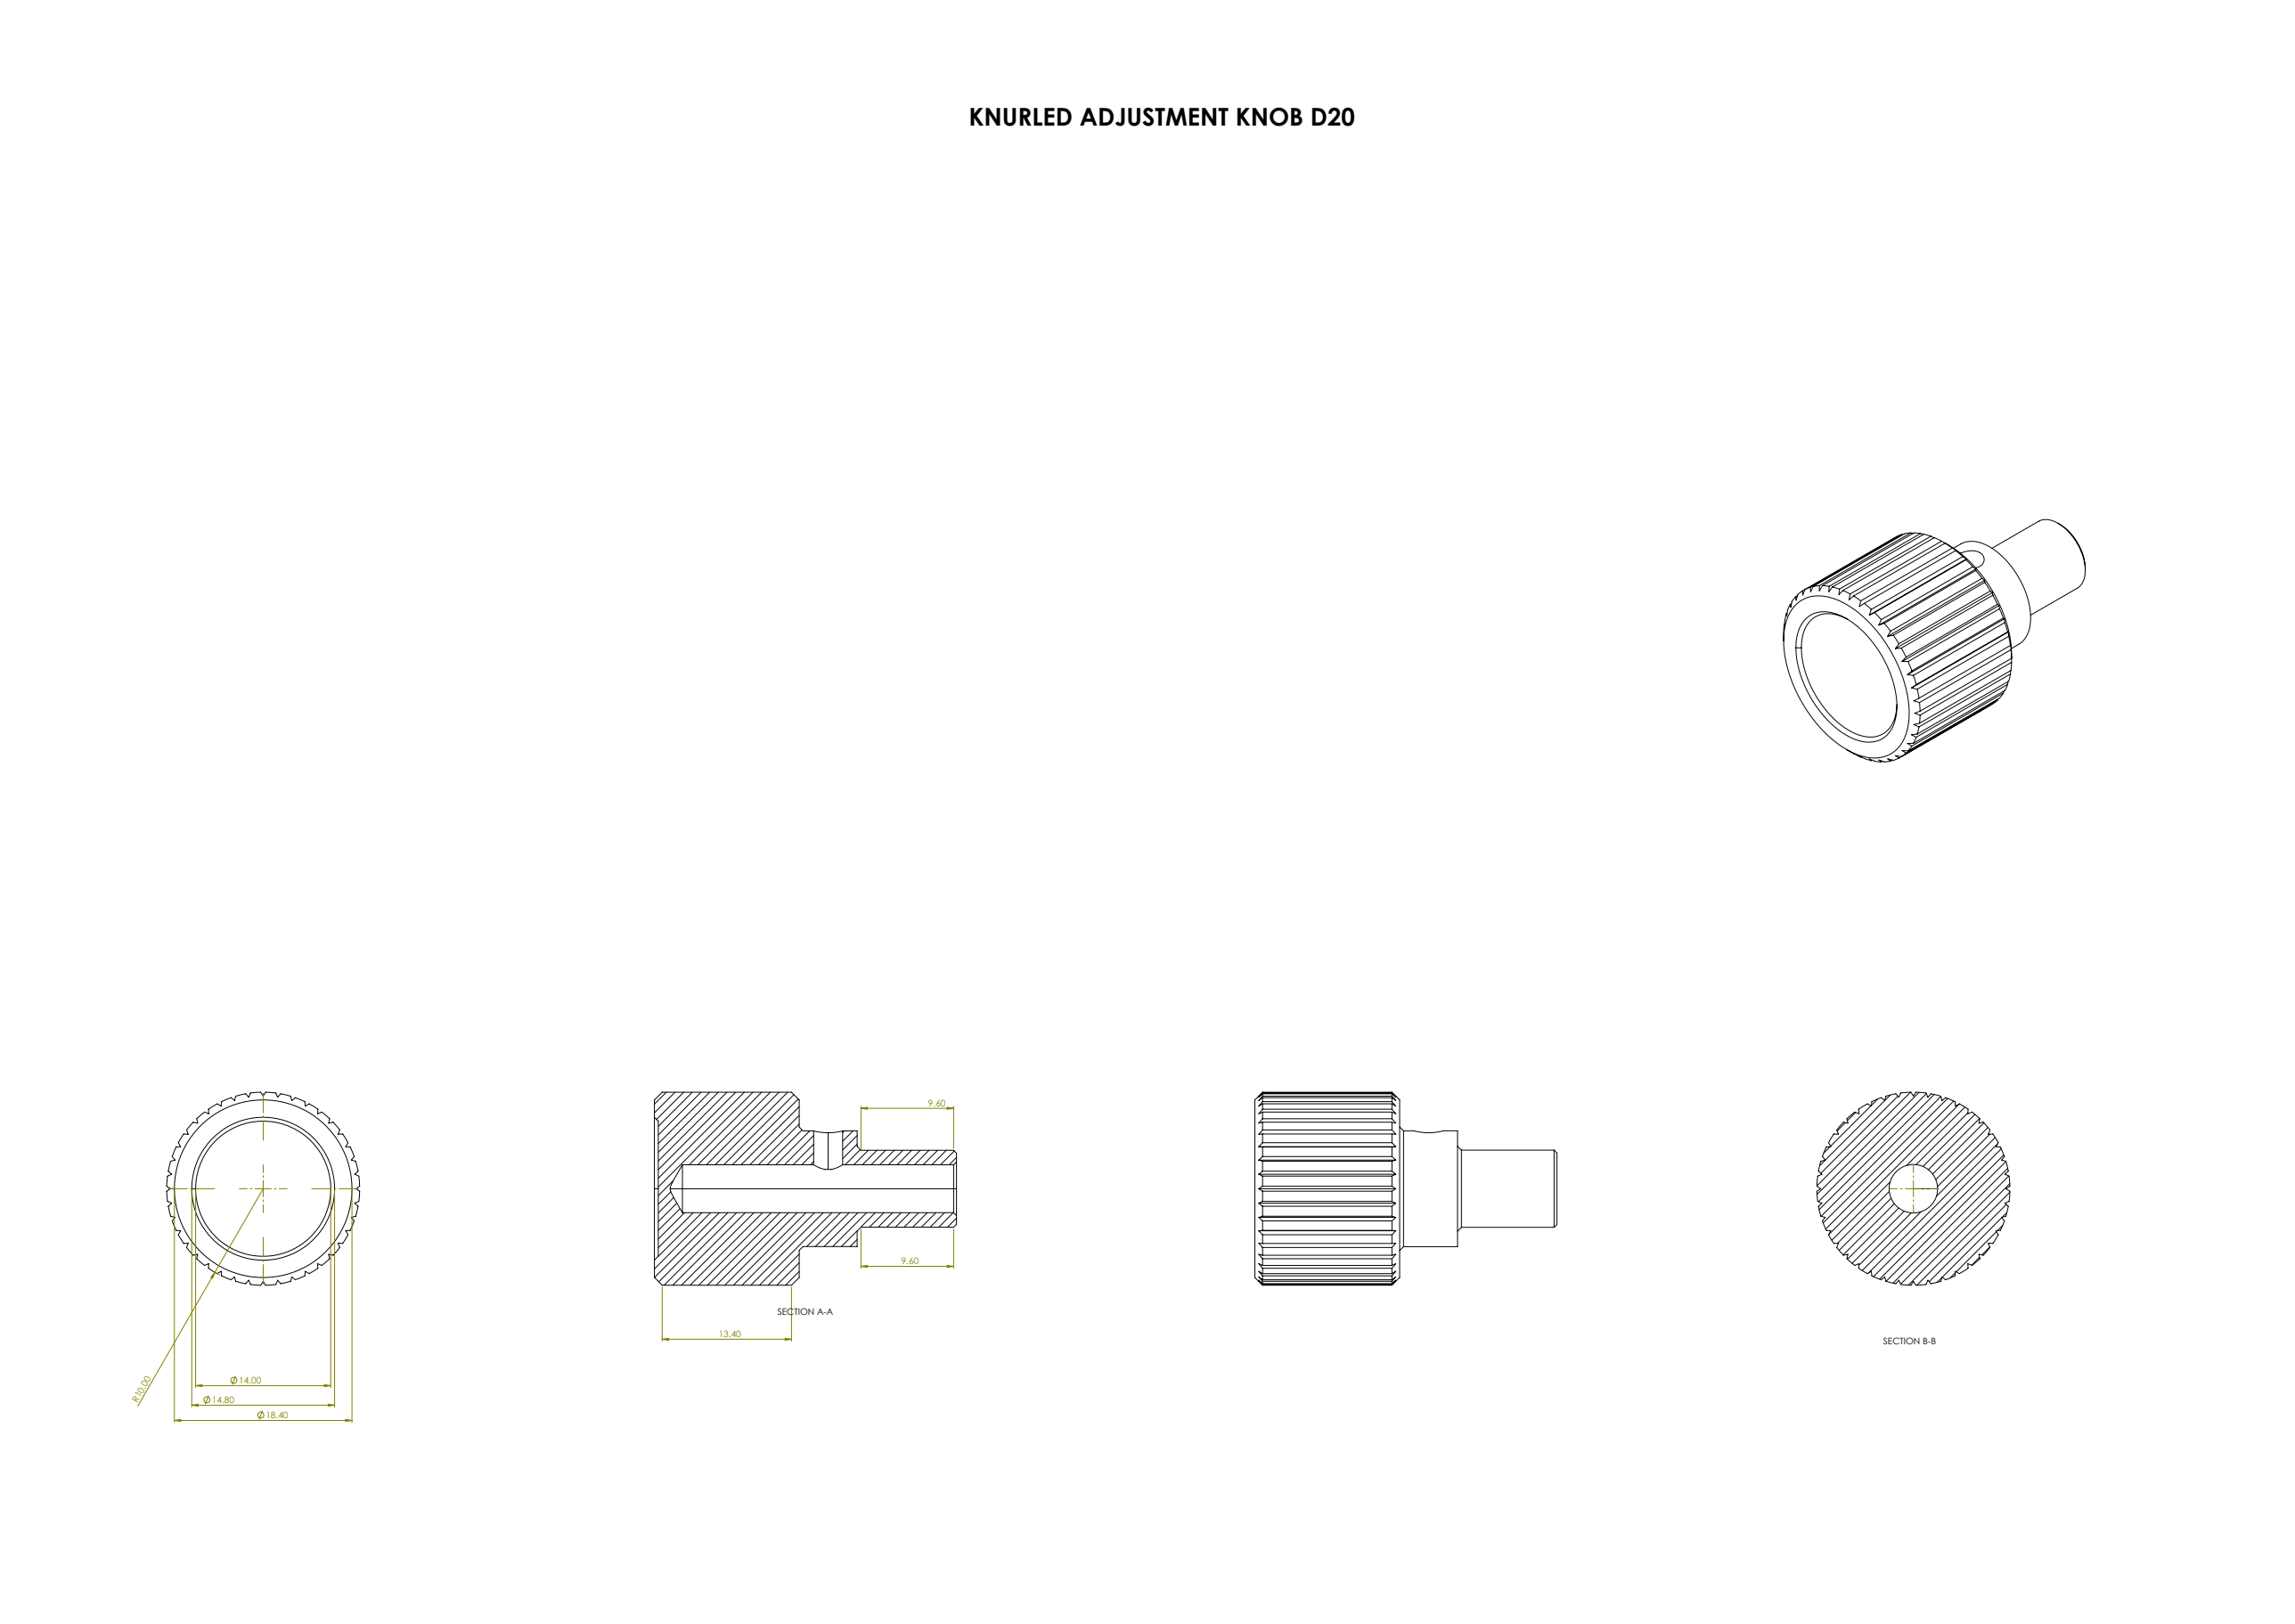
ISO-10303-21;
HEADER;
/* Generated by software containing ST-Developer
 * from STEP Tools, Inc. (www.steptools.com) 
 */

FILE_DESCRIPTION(
/* description */ (''),
/* implementation_level */ '2;1');

FILE_NAME(
/* name */ 'Knurled Adjustment Knob D20.step',
/* time_stamp */ '2026-10-05T09:57:53+05:00',
/* author */ (''),
/* organization */ (''),
/* preprocessor_version */ 'ST-DEVELOPER v20.2',
/* originating_system */ 'Autodesk Translation Framework v15.15.0.0',
/* authorisation */ '');

FILE_SCHEMA (('AUTOMOTIVE_DESIGN { 1 0 10303 214 3 1 1 }'));
ENDSEC;

DATA;
#10=MECHANICAL_DESIGN_GEOMETRIC_PRESENTATION_REPRESENTATION('',(#556),#113984);
#211=(
BOUNDED_CURVE()
B_SPLINE_CURVE(2,(#97814,#97815,#97816),.UNSPECIFIED.,.F.,.F.)
B_SPLINE_CURVE_WITH_KNOTS((3,3),(0.0639904841458714,0.1243156910283),
 .UNSPECIFIED.)
CURVE()
GEOMETRIC_REPRESENTATION_ITEM()
RATIONAL_B_SPLINE_CURVE((1.0006146198185,1.00059701757594,1.))
REPRESENTATION_ITEM('')
);
#212=(
BOUNDED_CURVE()
B_SPLINE_CURVE(2,(#97820,#97821,#97822),.UNSPECIFIED.,.F.,.F.)
B_SPLINE_CURVE_WITH_KNOTS((3,3),(0.,0.0603252068824429),.UNSPECIFIED.)
CURVE()
GEOMETRIC_REPRESENTATION_ITEM()
RATIONAL_B_SPLINE_CURVE((1.,1.00059701758504,1.00061461982786))
REPRESENTATION_ITEM('')
);
#213=(
BOUNDED_CURVE()
B_SPLINE_CURVE(2,(#97826,#97827,#97828),.UNSPECIFIED.,.F.,.F.)
B_SPLINE_CURVE_WITH_KNOTS((3,3),(0.,0.0603252068824511),.UNSPECIFIED.)
CURVE()
GEOMETRIC_REPRESENTATION_ITEM()
RATIONAL_B_SPLINE_CURVE((1.,1.00059701757207,1.00061461981452))
REPRESENTATION_ITEM('')
);
#214=(
BOUNDED_CURVE()
B_SPLINE_CURVE(2,(#97831,#97832,#97833),.UNSPECIFIED.,.F.,.F.)
B_SPLINE_CURVE_WITH_KNOTS((3,3),(0.0639904841458541,0.124315691028304),
 .UNSPECIFIED.)
CURVE()
GEOMETRIC_REPRESENTATION_ITEM()
RATIONAL_B_SPLINE_CURVE((1.00061461982307,1.00059701758038,1.))
REPRESENTATION_ITEM('')
);
#215=(
BOUNDED_CURVE()
B_SPLINE_CURVE(2,(#97838,#97839,#97840),.UNSPECIFIED.,.F.,.F.)
B_SPLINE_CURVE_WITH_KNOTS((3,3),(0.,0.0603252068825254),.UNSPECIFIED.)
CURVE()
GEOMETRIC_REPRESENTATION_ITEM()
RATIONAL_B_SPLINE_CURVE((1.,1.00059701756463,1.00061461980685))
REPRESENTATION_ITEM('')
);
#216=(
BOUNDED_CURVE()
B_SPLINE_CURVE(2,(#97842,#97843,#97844),.UNSPECIFIED.,.F.,.F.)
B_SPLINE_CURVE_WITH_KNOTS((3,3),(0.0639904841458276,0.124315691028306),
 .UNSPECIFIED.)
CURVE()
GEOMETRIC_REPRESENTATION_ITEM()
RATIONAL_B_SPLINE_CURVE((1.00061461981098,1.00059701756864,1.))
REPRESENTATION_ITEM('')
);
#217=(
BOUNDED_CURVE()
B_SPLINE_CURVE(2,(#97848,#97849,#97850),.UNSPECIFIED.,.F.,.F.)
B_SPLINE_CURVE_WITH_KNOTS((3,3),(0.,0.0603252068824394),.UNSPECIFIED.)
CURVE()
GEOMETRIC_REPRESENTATION_ITEM()
RATIONAL_B_SPLINE_CURVE((1.,1.00059701757103,1.00061461981344))
REPRESENTATION_ITEM('')
);
#218=(
BOUNDED_CURVE()
B_SPLINE_CURVE(2,(#97852,#97853,#97854),.UNSPECIFIED.,.F.,.F.)
B_SPLINE_CURVE_WITH_KNOTS((3,3),(0.0639904841458415,0.124315691028305),
 .UNSPECIFIED.)
CURVE()
GEOMETRIC_REPRESENTATION_ITEM()
RATIONAL_B_SPLINE_CURVE((1.00061461981036,1.00059701756804,1.))
REPRESENTATION_ITEM('')
);
#219=(
BOUNDED_CURVE()
B_SPLINE_CURVE(2,(#97858,#97859,#97860),.UNSPECIFIED.,.F.,.F.)
B_SPLINE_CURVE_WITH_KNOTS((3,3),(0.,0.0603252068825714),.UNSPECIFIED.)
CURVE()
GEOMETRIC_REPRESENTATION_ITEM()
RATIONAL_B_SPLINE_CURVE((1.,1.00059701757132,1.00061461981374))
REPRESENTATION_ITEM('')
);
#220=(
BOUNDED_CURVE()
B_SPLINE_CURVE(2,(#97862,#97863,#97864),.UNSPECIFIED.,.F.,.F.)
B_SPLINE_CURVE_WITH_KNOTS((3,3),(0.0639904841458359,0.124315691028304),
 .UNSPECIFIED.)
CURVE()
GEOMETRIC_REPRESENTATION_ITEM()
RATIONAL_B_SPLINE_CURVE((1.00061461982205,1.00059701757939,1.))
REPRESENTATION_ITEM('')
);
#221=(
BOUNDED_CURVE()
B_SPLINE_CURVE(2,(#97868,#97869,#97870),.UNSPECIFIED.,.F.,.F.)
B_SPLINE_CURVE_WITH_KNOTS((3,3),(0.,0.0603252068824456),.UNSPECIFIED.)
CURVE()
GEOMETRIC_REPRESENTATION_ITEM()
RATIONAL_B_SPLINE_CURVE((1.,1.00059701756571,1.00061461980796))
REPRESENTATION_ITEM('')
);
#222=(
BOUNDED_CURVE()
B_SPLINE_CURVE(2,(#97872,#97873,#97874),.UNSPECIFIED.,.F.,.F.)
B_SPLINE_CURVE_WITH_KNOTS((3,3),(0.0639904841458113,0.124315691028305),
 .UNSPECIFIED.)
CURVE()
GEOMETRIC_REPRESENTATION_ITEM()
RATIONAL_B_SPLINE_CURVE((1.00061461980765,1.00059701756541,1.))
REPRESENTATION_ITEM('')
);
#223=(
BOUNDED_CURVE()
B_SPLINE_CURVE(2,(#97878,#97879,#97880),.UNSPECIFIED.,.F.,.F.)
B_SPLINE_CURVE_WITH_KNOTS((3,3),(0.,0.0603252068824822),.UNSPECIFIED.)
CURVE()
GEOMETRIC_REPRESENTATION_ITEM()
RATIONAL_B_SPLINE_CURVE((1.,1.00059701756982,1.0006146198122))
REPRESENTATION_ITEM('')
);
#224=(
BOUNDED_CURVE()
B_SPLINE_CURVE(2,(#97882,#97883,#97884),.UNSPECIFIED.,.F.,.F.)
B_SPLINE_CURVE_WITH_KNOTS((3,3),(0.0639904841458351,0.124315691028304),
 .UNSPECIFIED.)
CURVE()
GEOMETRIC_REPRESENTATION_ITEM()
RATIONAL_B_SPLINE_CURVE((1.0006146198107,1.00059701756837,1.))
REPRESENTATION_ITEM('')
);
#225=(
BOUNDED_CURVE()
B_SPLINE_CURVE(2,(#97888,#97889,#97890),.UNSPECIFIED.,.F.,.F.)
B_SPLINE_CURVE_WITH_KNOTS((3,3),(0.,0.0603252068824583),.UNSPECIFIED.)
CURVE()
GEOMETRIC_REPRESENTATION_ITEM()
RATIONAL_B_SPLINE_CURVE((1.,1.00059701757041,1.0006146198128))
REPRESENTATION_ITEM('')
);
#226=(
BOUNDED_CURVE()
B_SPLINE_CURVE(2,(#97892,#97893,#97894),.UNSPECIFIED.,.F.,.F.)
B_SPLINE_CURVE_WITH_KNOTS((3,3),(0.0639904841458709,0.124315691028304),
 .UNSPECIFIED.)
CURVE()
GEOMETRIC_REPRESENTATION_ITEM()
RATIONAL_B_SPLINE_CURVE((1.00061461981124,1.00059701756889,1.))
REPRESENTATION_ITEM('')
);
#227=(
BOUNDED_CURVE()
B_SPLINE_CURVE(2,(#97898,#97899,#97900),.UNSPECIFIED.,.F.,.F.)
B_SPLINE_CURVE_WITH_KNOTS((3,3),(0.,0.0603252068824821),.UNSPECIFIED.)
CURVE()
GEOMETRIC_REPRESENTATION_ITEM()
RATIONAL_B_SPLINE_CURVE((1.,1.0005970175711,1.00061461981351))
REPRESENTATION_ITEM('')
);
#228=(
BOUNDED_CURVE()
B_SPLINE_CURVE(2,(#97902,#97903,#97904),.UNSPECIFIED.,.F.,.F.)
B_SPLINE_CURVE_WITH_KNOTS((3,3),(0.0639904841458647,0.124315691028304),
 .UNSPECIFIED.)
CURVE()
GEOMETRIC_REPRESENTATION_ITEM()
RATIONAL_B_SPLINE_CURVE((1.00061461981158,1.00059701756922,1.))
REPRESENTATION_ITEM('')
);
#229=(
BOUNDED_CURVE()
B_SPLINE_CURVE(2,(#97908,#97909,#97910),.UNSPECIFIED.,.F.,.F.)
B_SPLINE_CURVE_WITH_KNOTS((3,3),(0.,0.0603252068825191),.UNSPECIFIED.)
CURVE()
GEOMETRIC_REPRESENTATION_ITEM()
RATIONAL_B_SPLINE_CURVE((1.,1.00059701757121,1.00061461981363))
REPRESENTATION_ITEM('')
);
#230=(
BOUNDED_CURVE()
B_SPLINE_CURVE(2,(#97912,#97913,#97914),.UNSPECIFIED.,.F.,.F.)
B_SPLINE_CURVE_WITH_KNOTS((3,3),(0.063990484145815,0.124315691028306),
 .UNSPECIFIED.)
CURVE()
GEOMETRIC_REPRESENTATION_ITEM()
RATIONAL_B_SPLINE_CURVE((1.00061461981174,1.00059701756938,1.))
REPRESENTATION_ITEM('')
);
#231=(
BOUNDED_CURVE()
B_SPLINE_CURVE(2,(#97918,#97919,#97920),.UNSPECIFIED.,.F.,.F.)
B_SPLINE_CURVE_WITH_KNOTS((3,3),(0.,0.0603252068824783),.UNSPECIFIED.)
CURVE()
GEOMETRIC_REPRESENTATION_ITEM()
RATIONAL_B_SPLINE_CURVE((1.,1.00059701757256,1.00061461981502))
REPRESENTATION_ITEM('')
);
#232=(
BOUNDED_CURVE()
B_SPLINE_CURVE(2,(#97922,#97923,#97924),.UNSPECIFIED.,.F.,.F.)
B_SPLINE_CURVE_WITH_KNOTS((3,3),(0.0639904841458416,0.124315691028306),
 .UNSPECIFIED.)
CURVE()
GEOMETRIC_REPRESENTATION_ITEM()
RATIONAL_B_SPLINE_CURVE((1.00061461981231,1.00059701756993,1.))
REPRESENTATION_ITEM('')
);
#233=(
BOUNDED_CURVE()
B_SPLINE_CURVE(2,(#97928,#97929,#97930),.UNSPECIFIED.,.F.,.F.)
B_SPLINE_CURVE_WITH_KNOTS((3,3),(0.,0.0603252068824794),.UNSPECIFIED.)
CURVE()
GEOMETRIC_REPRESENTATION_ITEM()
RATIONAL_B_SPLINE_CURVE((1.,1.00059701756815,1.00061461981048))
REPRESENTATION_ITEM('')
);
#234=(
BOUNDED_CURVE()
B_SPLINE_CURVE(2,(#97932,#97933,#97934),.UNSPECIFIED.,.F.,.F.)
B_SPLINE_CURVE_WITH_KNOTS((3,3),(0.0639904841457963,0.124315691028306),
 .UNSPECIFIED.)
CURVE()
GEOMETRIC_REPRESENTATION_ITEM()
RATIONAL_B_SPLINE_CURVE((1.00061461981017,1.00059701756786,1.))
REPRESENTATION_ITEM('')
);
#235=(
BOUNDED_CURVE()
B_SPLINE_CURVE(2,(#97938,#97939,#97940),.UNSPECIFIED.,.F.,.F.)
B_SPLINE_CURVE_WITH_KNOTS((3,3),(0.,0.0603252068824883),.UNSPECIFIED.)
CURVE()
GEOMETRIC_REPRESENTATION_ITEM()
RATIONAL_B_SPLINE_CURVE((1.,1.00059701756951,1.00061461981188))
REPRESENTATION_ITEM('')
);
#236=(
BOUNDED_CURVE()
B_SPLINE_CURVE(2,(#97942,#97943,#97944),.UNSPECIFIED.,.F.,.F.)
B_SPLINE_CURVE_WITH_KNOTS((3,3),(0.0639904841458018,0.124315691028305),
 .UNSPECIFIED.)
CURVE()
GEOMETRIC_REPRESENTATION_ITEM()
RATIONAL_B_SPLINE_CURVE((1.00061461980912,1.00059701756684,1.))
REPRESENTATION_ITEM('')
);
#237=(
BOUNDED_CURVE()
B_SPLINE_CURVE(2,(#97948,#97949,#97950),.UNSPECIFIED.,.F.,.F.)
B_SPLINE_CURVE_WITH_KNOTS((3,3),(0.,0.0603252068824852),.UNSPECIFIED.)
CURVE()
GEOMETRIC_REPRESENTATION_ITEM()
RATIONAL_B_SPLINE_CURVE((1.,1.00059701756809,1.00061461981042))
REPRESENTATION_ITEM('')
);
#238=(
BOUNDED_CURVE()
B_SPLINE_CURVE(2,(#97952,#97953,#97954),.UNSPECIFIED.,.F.,.F.)
B_SPLINE_CURVE_WITH_KNOTS((3,3),(0.0639904841458453,0.124315691028304),
 .UNSPECIFIED.)
CURVE()
GEOMETRIC_REPRESENTATION_ITEM()
RATIONAL_B_SPLINE_CURVE((1.0006146198128,1.00059701757041,1.))
REPRESENTATION_ITEM('')
);
#239=(
BOUNDED_CURVE()
B_SPLINE_CURVE(2,(#97958,#97959,#97960),.UNSPECIFIED.,.F.,.F.)
B_SPLINE_CURVE_WITH_KNOTS((3,3),(0.,0.06032520688249),.UNSPECIFIED.)
CURVE()
GEOMETRIC_REPRESENTATION_ITEM()
RATIONAL_B_SPLINE_CURVE((1.,1.00059701756971,1.00061461981208))
REPRESENTATION_ITEM('')
);
#240=(
BOUNDED_CURVE()
B_SPLINE_CURVE(2,(#97962,#97963,#97964),.UNSPECIFIED.,.F.,.F.)
B_SPLINE_CURVE_WITH_KNOTS((3,3),(0.0639904841458239,0.124315691028304),
 .UNSPECIFIED.)
CURVE()
GEOMETRIC_REPRESENTATION_ITEM()
RATIONAL_B_SPLINE_CURVE((1.0006146198114,1.00059701756905,1.))
REPRESENTATION_ITEM('')
);
#241=(
BOUNDED_CURVE()
B_SPLINE_CURVE(2,(#97968,#97969,#97970),.UNSPECIFIED.,.F.,.F.)
B_SPLINE_CURVE_WITH_KNOTS((3,3),(0.,0.0603252068824721),.UNSPECIFIED.)
CURVE()
GEOMETRIC_REPRESENTATION_ITEM()
RATIONAL_B_SPLINE_CURVE((1.,1.0005970175654,1.00061461980764))
REPRESENTATION_ITEM('')
);
#242=(
BOUNDED_CURVE()
B_SPLINE_CURVE(2,(#97972,#97973,#97974),.UNSPECIFIED.,.F.,.F.)
B_SPLINE_CURVE_WITH_KNOTS((3,3),(0.0639904841458158,0.124315691028305),
 .UNSPECIFIED.)
CURVE()
GEOMETRIC_REPRESENTATION_ITEM()
RATIONAL_B_SPLINE_CURVE((1.00061461980759,1.00059701756535,1.))
REPRESENTATION_ITEM('')
);
#243=(
BOUNDED_CURVE()
B_SPLINE_CURVE(2,(#97978,#97979,#97980),.UNSPECIFIED.,.F.,.F.)
B_SPLINE_CURVE_WITH_KNOTS((3,3),(0.,0.0603252068824717),.UNSPECIFIED.)
CURVE()
GEOMETRIC_REPRESENTATION_ITEM()
RATIONAL_B_SPLINE_CURVE((1.,1.00059701757901,1.00061461982166))
REPRESENTATION_ITEM('')
);
#244=(
BOUNDED_CURVE()
B_SPLINE_CURVE(2,(#97982,#97983,#97984),.UNSPECIFIED.,.F.,.F.)
B_SPLINE_CURVE_WITH_KNOTS((3,3),(0.063990484145796,0.124315691028302),
 .UNSPECIFIED.)
CURVE()
GEOMETRIC_REPRESENTATION_ITEM()
RATIONAL_B_SPLINE_CURVE((1.0006146198112,1.00059701756885,1.))
REPRESENTATION_ITEM('')
);
#245=(
BOUNDED_CURVE()
B_SPLINE_CURVE(2,(#97988,#97989,#97990),.UNSPECIFIED.,.F.,.F.)
B_SPLINE_CURVE_WITH_KNOTS((3,3),(0.,0.0603252068824572),.UNSPECIFIED.)
CURVE()
GEOMETRIC_REPRESENTATION_ITEM()
RATIONAL_B_SPLINE_CURVE((1.,1.00059701757014,1.00061461981252))
REPRESENTATION_ITEM('')
);
#246=(
BOUNDED_CURVE()
B_SPLINE_CURVE(2,(#97992,#97993,#97994),.UNSPECIFIED.,.F.,.F.)
B_SPLINE_CURVE_WITH_KNOTS((3,3),(0.0639904841458277,0.124315691028304),
 .UNSPECIFIED.)
CURVE()
GEOMETRIC_REPRESENTATION_ITEM()
RATIONAL_B_SPLINE_CURVE((1.00061461981263,1.00059701757024,1.))
REPRESENTATION_ITEM('')
);
#247=(
BOUNDED_CURVE()
B_SPLINE_CURVE(2,(#97998,#97999,#98000),.UNSPECIFIED.,.F.,.F.)
B_SPLINE_CURVE_WITH_KNOTS((3,3),(0.,0.0603252068824675),.UNSPECIFIED.)
CURVE()
GEOMETRIC_REPRESENTATION_ITEM()
RATIONAL_B_SPLINE_CURVE((1.,1.00059701756283,1.000614619805))
REPRESENTATION_ITEM('')
);
#248=(
BOUNDED_CURVE()
B_SPLINE_CURVE(2,(#98002,#98003,#98004),.UNSPECIFIED.,.F.,.F.)
B_SPLINE_CURVE_WITH_KNOTS((3,3),(0.0639904841458849,0.124315691028304),
 .UNSPECIFIED.)
CURVE()
GEOMETRIC_REPRESENTATION_ITEM()
RATIONAL_B_SPLINE_CURVE((1.00061461981573,1.00059701757326,1.))
REPRESENTATION_ITEM('')
);
#249=(
BOUNDED_CURVE()
B_SPLINE_CURVE(2,(#98008,#98009,#98010),.UNSPECIFIED.,.F.,.F.)
B_SPLINE_CURVE_WITH_KNOTS((3,3),(0.,0.0603252068824598),.UNSPECIFIED.)
CURVE()
GEOMETRIC_REPRESENTATION_ITEM()
RATIONAL_B_SPLINE_CURVE((1.,1.0005970175702,1.00061461981259))
REPRESENTATION_ITEM('')
);
#250=(
BOUNDED_CURVE()
B_SPLINE_CURVE(2,(#98012,#98013,#98014),.UNSPECIFIED.,.F.,.F.)
B_SPLINE_CURVE_WITH_KNOTS((3,3),(0.0639904841458239,0.124315691028304),
 .UNSPECIFIED.)
CURVE()
GEOMETRIC_REPRESENTATION_ITEM()
RATIONAL_B_SPLINE_CURVE((1.00061461981594,1.00059701757346,1.))
REPRESENTATION_ITEM('')
);
#251=(
BOUNDED_CURVE()
B_SPLINE_CURVE(2,(#98018,#98019,#98020),.UNSPECIFIED.,.F.,.F.)
B_SPLINE_CURVE_WITH_KNOTS((3,3),(0.,0.0603252068824849),.UNSPECIFIED.)
CURVE()
GEOMETRIC_REPRESENTATION_ITEM()
RATIONAL_B_SPLINE_CURVE((1.,1.00059701756587,1.00061461980812))
REPRESENTATION_ITEM('')
);
#252=(
BOUNDED_CURVE()
B_SPLINE_CURVE(2,(#98025,#98026,#98027),.UNSPECIFIED.,.F.,.F.)
B_SPLINE_CURVE_WITH_KNOTS((3,3),(0.0639904841458217,0.124315691028305),
 .UNSPECIFIED.)
CURVE()
GEOMETRIC_REPRESENTATION_ITEM()
RATIONAL_B_SPLINE_CURVE((1.00061461980612,1.00059701756392,1.))
REPRESENTATION_ITEM('')
);
#253=(
BOUNDED_CURVE()
B_SPLINE_CURVE(2,(#98031,#98032,#98033),.UNSPECIFIED.,.F.,.F.)
B_SPLINE_CURVE_WITH_KNOTS((3,3),(0.,0.060325206882456),.UNSPECIFIED.)
CURVE()
GEOMETRIC_REPRESENTATION_ITEM()
RATIONAL_B_SPLINE_CURVE((1.,1.00059701757113,1.00061461981354))
REPRESENTATION_ITEM('')
);
#254=(
BOUNDED_CURVE()
B_SPLINE_CURVE(2,(#98035,#98036,#98037),.UNSPECIFIED.,.F.,.F.)
B_SPLINE_CURVE_WITH_KNOTS((3,3),(0.0639904841458245,0.124315691028306),
 .UNSPECIFIED.)
CURVE()
GEOMETRIC_REPRESENTATION_ITEM()
RATIONAL_B_SPLINE_CURVE((1.00061461981538,1.00059701757292,1.))
REPRESENTATION_ITEM('')
);
#255=(
BOUNDED_CURVE()
B_SPLINE_CURVE(2,(#98041,#98042,#98043),.UNSPECIFIED.,.F.,.F.)
B_SPLINE_CURVE_WITH_KNOTS((3,3),(0.,0.0603252068824492),.UNSPECIFIED.)
CURVE()
GEOMETRIC_REPRESENTATION_ITEM()
RATIONAL_B_SPLINE_CURVE((1.,1.0005970175686,1.00061461981094))
REPRESENTATION_ITEM('')
);
#256=(
BOUNDED_CURVE()
B_SPLINE_CURVE(2,(#98045,#98046,#98047),.UNSPECIFIED.,.F.,.F.)
B_SPLINE_CURVE_WITH_KNOTS((3,3),(0.0639904841457976,0.124315691028306),
 .UNSPECIFIED.)
CURVE()
GEOMETRIC_REPRESENTATION_ITEM()
RATIONAL_B_SPLINE_CURVE((1.00061461981101,1.00059701756867,1.))
REPRESENTATION_ITEM('')
);
#257=(
BOUNDED_CURVE()
B_SPLINE_CURVE(2,(#98051,#98052,#98053),.UNSPECIFIED.,.F.,.F.)
B_SPLINE_CURVE_WITH_KNOTS((3,3),(0.,0.0603252068824974),.UNSPECIFIED.)
CURVE()
GEOMETRIC_REPRESENTATION_ITEM()
RATIONAL_B_SPLINE_CURVE((1.,1.00059701757075,1.00061461981315))
REPRESENTATION_ITEM('')
);
#258=(
BOUNDED_CURVE()
B_SPLINE_CURVE(2,(#98055,#98056,#98057),.UNSPECIFIED.,.F.,.F.)
B_SPLINE_CURVE_WITH_KNOTS((3,3),(0.0639904841458211,0.124315691028304),
 .UNSPECIFIED.)
CURVE()
GEOMETRIC_REPRESENTATION_ITEM()
RATIONAL_B_SPLINE_CURVE((1.00061461981339,1.00059701757099,1.))
REPRESENTATION_ITEM('')
);
#259=(
BOUNDED_CURVE()
B_SPLINE_CURVE(2,(#98061,#98062,#98063),.UNSPECIFIED.,.F.,.F.)
B_SPLINE_CURVE_WITH_KNOTS((3,3),(0.,0.0603252068824656),.UNSPECIFIED.)
CURVE()
GEOMETRIC_REPRESENTATION_ITEM()
RATIONAL_B_SPLINE_CURVE((1.,1.00059701757014,1.00061461981252))
REPRESENTATION_ITEM('')
);
#260=(
BOUNDED_CURVE()
B_SPLINE_CURVE(2,(#98065,#98066,#98067),.UNSPECIFIED.,.F.,.F.)
B_SPLINE_CURVE_WITH_KNOTS((3,3),(0.0639904841457857,0.124315691028306),
 .UNSPECIFIED.)
CURVE()
GEOMETRIC_REPRESENTATION_ITEM()
RATIONAL_B_SPLINE_CURVE((1.00061461980911,1.00059701756683,1.))
REPRESENTATION_ITEM('')
);
#261=(
BOUNDED_CURVE()
B_SPLINE_CURVE(2,(#98071,#98072,#98073),.UNSPECIFIED.,.F.,.F.)
B_SPLINE_CURVE_WITH_KNOTS((3,3),(0.,0.0603252068825302),.UNSPECIFIED.)
CURVE()
GEOMETRIC_REPRESENTATION_ITEM()
RATIONAL_B_SPLINE_CURVE((1.,1.00059701756736,1.00061461980966))
REPRESENTATION_ITEM('')
);
#262=(
BOUNDED_CURVE()
B_SPLINE_CURVE(2,(#98075,#98076,#98077),.UNSPECIFIED.,.F.,.F.)
B_SPLINE_CURVE_WITH_KNOTS((3,3),(0.0639904841458149,0.124315691028305),
 .UNSPECIFIED.)
CURVE()
GEOMETRIC_REPRESENTATION_ITEM()
RATIONAL_B_SPLINE_CURVE((1.00061461980823,1.00059701756597,1.))
REPRESENTATION_ITEM('')
);
#263=(
BOUNDED_CURVE()
B_SPLINE_CURVE(2,(#98081,#98082,#98083),.UNSPECIFIED.,.F.,.F.)
B_SPLINE_CURVE_WITH_KNOTS((3,3),(0.,0.0603252068825094),.UNSPECIFIED.)
CURVE()
GEOMETRIC_REPRESENTATION_ITEM()
RATIONAL_B_SPLINE_CURVE((1.,1.00059701757625,1.00061461981881))
REPRESENTATION_ITEM('')
);
#264=(
BOUNDED_CURVE()
B_SPLINE_CURVE(2,(#98085,#98086,#98087),.UNSPECIFIED.,.F.,.F.)
B_SPLINE_CURVE_WITH_KNOTS((3,3),(0.0639904841458013,0.124315691028303),
 .UNSPECIFIED.)
CURVE()
GEOMETRIC_REPRESENTATION_ITEM()
RATIONAL_B_SPLINE_CURVE((1.00061461981526,1.0005970175728,1.))
REPRESENTATION_ITEM('')
);
#265=(
BOUNDED_CURVE()
B_SPLINE_CURVE(2,(#98091,#98092,#98093),.UNSPECIFIED.,.F.,.F.)
B_SPLINE_CURVE_WITH_KNOTS((3,3),(0.,0.060325206882548),.UNSPECIFIED.)
CURVE()
GEOMETRIC_REPRESENTATION_ITEM()
RATIONAL_B_SPLINE_CURVE((1.,1.0005970175677,1.00061461981001))
REPRESENTATION_ITEM('')
);
#266=(
BOUNDED_CURVE()
B_SPLINE_CURVE(2,(#98095,#98096,#98097),.UNSPECIFIED.,.F.,.F.)
B_SPLINE_CURVE_WITH_KNOTS((3,3),(0.0639904841458135,0.124315691028304),
 .UNSPECIFIED.)
CURVE()
GEOMETRIC_REPRESENTATION_ITEM()
RATIONAL_B_SPLINE_CURVE((1.00061461981065,1.00059701756832,1.))
REPRESENTATION_ITEM('')
);
#267=(
BOUNDED_CURVE()
B_SPLINE_CURVE(2,(#98101,#98102,#98103),.UNSPECIFIED.,.F.,.F.)
B_SPLINE_CURVE_WITH_KNOTS((3,3),(0.,0.0603252068824779),.UNSPECIFIED.)
CURVE()
GEOMETRIC_REPRESENTATION_ITEM()
RATIONAL_B_SPLINE_CURVE((1.,1.00059701756951,1.00061461981188))
REPRESENTATION_ITEM('')
);
#268=(
BOUNDED_CURVE()
B_SPLINE_CURVE(2,(#98105,#98106,#98107),.UNSPECIFIED.,.F.,.F.)
B_SPLINE_CURVE_WITH_KNOTS((3,3),(0.0639904841458649,0.124315691028304),
 .UNSPECIFIED.)
CURVE()
GEOMETRIC_REPRESENTATION_ITEM()
RATIONAL_B_SPLINE_CURVE((1.00061461981009,1.00059701756778,1.))
REPRESENTATION_ITEM('')
);
#269=(
BOUNDED_CURVE()
B_SPLINE_CURVE(2,(#98111,#98112,#98113),.UNSPECIFIED.,.F.,.F.)
B_SPLINE_CURVE_WITH_KNOTS((3,3),(0.,0.0603252068824628),.UNSPECIFIED.)
CURVE()
GEOMETRIC_REPRESENTATION_ITEM()
RATIONAL_B_SPLINE_CURVE((1.,1.00059701757151,1.00061461981393))
REPRESENTATION_ITEM('')
);
#270=(
BOUNDED_CURVE()
B_SPLINE_CURVE(2,(#98115,#98116,#98117),.UNSPECIFIED.,.F.,.F.)
B_SPLINE_CURVE_WITH_KNOTS((3,3),(0.0639904841458699,0.124315691028302),
 .UNSPECIFIED.)
CURVE()
GEOMETRIC_REPRESENTATION_ITEM()
RATIONAL_B_SPLINE_CURVE((1.000614619814,1.00059701757158,1.))
REPRESENTATION_ITEM('')
);
#271=(
BOUNDED_CURVE()
B_SPLINE_CURVE(2,(#98121,#98122,#98123),.UNSPECIFIED.,.F.,.F.)
B_SPLINE_CURVE_WITH_KNOTS((3,3),(0.,0.0603252068824368),.UNSPECIFIED.)
CURVE()
GEOMETRIC_REPRESENTATION_ITEM()
RATIONAL_B_SPLINE_CURVE((1.,1.00059701757288,1.00061461981535))
REPRESENTATION_ITEM('')
);
#272=(
BOUNDED_CURVE()
B_SPLINE_CURVE(2,(#98125,#98126,#98127),.UNSPECIFIED.,.F.,.F.)
B_SPLINE_CURVE_WITH_KNOTS((3,3),(0.0639904841458755,0.124315691028302),
 .UNSPECIFIED.)
CURVE()
GEOMETRIC_REPRESENTATION_ITEM()
RATIONAL_B_SPLINE_CURVE((1.00061461981817,1.00059701757562,1.))
REPRESENTATION_ITEM('')
);
#273=(
BOUNDED_CURVE()
B_SPLINE_CURVE(2,(#98131,#98132,#98133),.UNSPECIFIED.,.F.,.F.)
B_SPLINE_CURVE_WITH_KNOTS((3,3),(0.,0.0603252068823799),.UNSPECIFIED.)
CURVE()
GEOMETRIC_REPRESENTATION_ITEM()
RATIONAL_B_SPLINE_CURVE((1.,1.00059701757321,1.00061461981569))
REPRESENTATION_ITEM('')
);
#274=(
BOUNDED_CURVE()
B_SPLINE_CURVE(2,(#98135,#98136,#98137),.UNSPECIFIED.,.F.,.F.)
B_SPLINE_CURVE_WITH_KNOTS((3,3),(0.0639904841458814,0.1243156910283),
 .UNSPECIFIED.)
CURVE()
GEOMETRIC_REPRESENTATION_ITEM()
RATIONAL_B_SPLINE_CURVE((1.00061461981777,1.00059701757523,1.))
REPRESENTATION_ITEM('')
);
#275=(
BOUNDED_CURVE()
B_SPLINE_CURVE(2,(#98141,#98142,#98143),.UNSPECIFIED.,.F.,.F.)
B_SPLINE_CURVE_WITH_KNOTS((3,3),(0.,0.0603252068824466),.UNSPECIFIED.)
CURVE()
GEOMETRIC_REPRESENTATION_ITEM()
RATIONAL_B_SPLINE_CURVE((1.,1.0005970175777,1.00061461982031))
REPRESENTATION_ITEM('')
);
#276=(
BOUNDED_CURVE()
B_SPLINE_CURVE(2,(#98145,#98146,#98147),.UNSPECIFIED.,.F.,.F.)
B_SPLINE_CURVE_WITH_KNOTS((3,3),(0.0639904841458398,0.124315691028299),
 .UNSPECIFIED.)
CURVE()
GEOMETRIC_REPRESENTATION_ITEM()
RATIONAL_B_SPLINE_CURVE((1.00061461981638,1.00059701757389,1.))
REPRESENTATION_ITEM('')
);
#277=(
BOUNDED_CURVE()
B_SPLINE_CURVE(2,(#98151,#98152,#98153),.UNSPECIFIED.,.F.,.F.)
B_SPLINE_CURVE_WITH_KNOTS((3,3),(0.,0.06032520688241),.UNSPECIFIED.)
CURVE()
GEOMETRIC_REPRESENTATION_ITEM()
RATIONAL_B_SPLINE_CURVE((1.,1.00059701757236,1.00061461981481))
REPRESENTATION_ITEM('')
);
#278=(
BOUNDED_CURVE()
B_SPLINE_CURVE(2,(#98155,#98156,#98157),.UNSPECIFIED.,.F.,.F.)
B_SPLINE_CURVE_WITH_KNOTS((3,3),(0.0639904841458318,0.124315691028302),
 .UNSPECIFIED.)
CURVE()
GEOMETRIC_REPRESENTATION_ITEM()
RATIONAL_B_SPLINE_CURVE((1.00061461981596,1.00059701757347,1.))
REPRESENTATION_ITEM('')
);
#279=(
BOUNDED_CURVE()
B_SPLINE_CURVE(2,(#98161,#98162,#98163),.UNSPECIFIED.,.F.,.F.)
B_SPLINE_CURVE_WITH_KNOTS((3,3),(0.,0.0603252068823898),.UNSPECIFIED.)
CURVE()
GEOMETRIC_REPRESENTATION_ITEM()
RATIONAL_B_SPLINE_CURVE((1.,1.00059701757645,1.00061461981902))
REPRESENTATION_ITEM('')
);
#280=(
BOUNDED_CURVE()
B_SPLINE_CURVE(2,(#98165,#98166,#98167),.UNSPECIFIED.,.F.,.F.)
B_SPLINE_CURVE_WITH_KNOTS((3,3),(0.0639904841459118,0.1243156910283),
 .UNSPECIFIED.)
CURVE()
GEOMETRIC_REPRESENTATION_ITEM()
RATIONAL_B_SPLINE_CURVE((1.00061461981901,1.00059701757644,1.))
REPRESENTATION_ITEM('')
);
#281=(
BOUNDED_CURVE()
B_SPLINE_CURVE(2,(#98171,#98172,#98173),.UNSPECIFIED.,.F.,.F.)
B_SPLINE_CURVE_WITH_KNOTS((3,3),(0.,0.0603252068824294),.UNSPECIFIED.)
CURVE()
GEOMETRIC_REPRESENTATION_ITEM()
RATIONAL_B_SPLINE_CURVE((1.,1.00059701757539,1.00061461981793))
REPRESENTATION_ITEM('')
);
#282=(
BOUNDED_CURVE()
B_SPLINE_CURVE(2,(#98175,#98176,#98177),.UNSPECIFIED.,.F.,.F.)
B_SPLINE_CURVE_WITH_KNOTS((3,3),(0.0639904841458455,0.1243156910283),
 .UNSPECIFIED.)
CURVE()
GEOMETRIC_REPRESENTATION_ITEM()
RATIONAL_B_SPLINE_CURVE((1.00061461982149,1.00059701757885,1.))
REPRESENTATION_ITEM('')
);
#283=(
BOUNDED_CURVE()
B_SPLINE_CURVE(2,(#98181,#98182,#98183),.UNSPECIFIED.,.F.,.F.)
B_SPLINE_CURVE_WITH_KNOTS((3,3),(0.,0.0603252068824333),.UNSPECIFIED.)
CURVE()
GEOMETRIC_REPRESENTATION_ITEM()
RATIONAL_B_SPLINE_CURVE((1.,1.00059701757328,1.00061461981575))
REPRESENTATION_ITEM('')
);
#284=(
BOUNDED_CURVE()
B_SPLINE_CURVE(2,(#98185,#98186,#98187),.UNSPECIFIED.,.F.,.F.)
B_SPLINE_CURVE_WITH_KNOTS((3,3),(0.0639904841458647,0.124315691028299),
 .UNSPECIFIED.)
CURVE()
GEOMETRIC_REPRESENTATION_ITEM()
RATIONAL_B_SPLINE_CURVE((1.00061461981117,1.00059701756882,1.))
REPRESENTATION_ITEM('')
);
#285=(
BOUNDED_CURVE()
B_SPLINE_CURVE(2,(#98191,#98192,#98193),.UNSPECIFIED.,.F.,.F.)
B_SPLINE_CURVE_WITH_KNOTS((3,3),(0.,0.060325206882429),.UNSPECIFIED.)
CURVE()
GEOMETRIC_REPRESENTATION_ITEM()
RATIONAL_B_SPLINE_CURVE((1.,1.00059701757149,1.00061461981392))
REPRESENTATION_ITEM('')
);
#286=(
BOUNDED_CURVE()
B_SPLINE_CURVE(2,(#98195,#98196,#98197),.UNSPECIFIED.,.F.,.F.)
B_SPLINE_CURVE_WITH_KNOTS((3,3),(0.0639904841459033,0.1243156910283),
 .UNSPECIFIED.)
CURVE()
GEOMETRIC_REPRESENTATION_ITEM()
RATIONAL_B_SPLINE_CURVE((1.00061461981837,1.00059701757582,1.))
REPRESENTATION_ITEM('')
);
#287=(
BOUNDED_CURVE()
B_SPLINE_CURVE(2,(#98201,#98202,#98203),.UNSPECIFIED.,.F.,.F.)
B_SPLINE_CURVE_WITH_KNOTS((3,3),(0.,0.0603252068824625),.UNSPECIFIED.)
CURVE()
GEOMETRIC_REPRESENTATION_ITEM()
RATIONAL_B_SPLINE_CURVE((1.,1.00059701757607,1.00061461981863))
REPRESENTATION_ITEM('')
);
#288=(
BOUNDED_CURVE()
B_SPLINE_CURVE(2,(#98205,#98206,#98207),.UNSPECIFIED.,.F.,.F.)
B_SPLINE_CURVE_WITH_KNOTS((3,3),(0.0639904841458564,0.124315691028299),
 .UNSPECIFIED.)
CURVE()
GEOMETRIC_REPRESENTATION_ITEM()
RATIONAL_B_SPLINE_CURVE((1.00061461981741,1.00059701757488,1.))
REPRESENTATION_ITEM('')
);
#289=(
BOUNDED_CURVE()
B_SPLINE_CURVE(2,(#98211,#98212,#98213),.UNSPECIFIED.,.F.,.F.)
B_SPLINE_CURVE_WITH_KNOTS((3,3),(0.,0.0603252068824167),.UNSPECIFIED.)
CURVE()
GEOMETRIC_REPRESENTATION_ITEM()
RATIONAL_B_SPLINE_CURVE((1.,1.00059701757614,1.0006146198187))
REPRESENTATION_ITEM('')
);
#290=(
BOUNDED_CURVE()
B_SPLINE_CURVE(2,(#98215,#98216,#98217),.UNSPECIFIED.,.F.,.F.)
B_SPLINE_CURVE_WITH_KNOTS((3,3),(0.0639904841458993,0.1243156910283),
 .UNSPECIFIED.)
CURVE()
GEOMETRIC_REPRESENTATION_ITEM()
RATIONAL_B_SPLINE_CURVE((1.00061461981727,1.00059701757475,1.))
REPRESENTATION_ITEM('')
);
#291=(
BOUNDED_CURVE()
B_SPLINE_CURVE(2,(#98221,#98222,#98223),.UNSPECIFIED.,.F.,.F.)
B_SPLINE_CURVE_WITH_KNOTS((3,3),(0.,0.0603252068824493),.UNSPECIFIED.)
CURVE()
GEOMETRIC_REPRESENTATION_ITEM()
RATIONAL_B_SPLINE_CURVE((1.,1.00059701757429,1.00061461981679))
REPRESENTATION_ITEM('')
);
#292=(
BOUNDED_CURVE()
B_SPLINE_CURVE(2,(#98225,#98226,#98227),.UNSPECIFIED.,.F.,.F.)
B_SPLINE_CURVE_WITH_KNOTS((3,3),(0.0639904841458732,0.124315691028301),
 .UNSPECIFIED.)
CURVE()
GEOMETRIC_REPRESENTATION_ITEM()
RATIONAL_B_SPLINE_CURVE((1.00061461981735,1.00059701757483,1.))
REPRESENTATION_ITEM('')
);
#293=(
BOUNDED_CURVE()
B_SPLINE_CURVE(2,(#98241,#98242,#98243),.UNSPECIFIED.,.F.,.F.)
B_SPLINE_CURVE_WITH_KNOTS((3,3),(0.,0.0603252068824331),.UNSPECIFIED.)
CURVE()
GEOMETRIC_REPRESENTATION_ITEM()
RATIONAL_B_SPLINE_CURVE((1.,1.00059701757411,1.00061461981661))
REPRESENTATION_ITEM('')
);
#294=(
BOUNDED_CURVE()
B_SPLINE_CURVE(2,(#98246,#98247,#98248),.UNSPECIFIED.,.F.,.F.)
B_SPLINE_CURVE_WITH_KNOTS((3,3),(0.0639904841458569,0.124315691028302),
 .UNSPECIFIED.)
CURVE()
GEOMETRIC_REPRESENTATION_ITEM()
RATIONAL_B_SPLINE_CURVE((1.00061461981636,1.00059701757387,1.))
REPRESENTATION_ITEM('')
);
#295=(
BOUNDED_CURVE()
B_SPLINE_CURVE(2,(#98259,#98260,#98261),.UNSPECIFIED.,.F.,.F.)
B_SPLINE_CURVE_WITH_KNOTS((3,3),(0.0639904841458384,0.124315691028303),
 .UNSPECIFIED.)
CURVE()
GEOMETRIC_REPRESENTATION_ITEM()
RATIONAL_B_SPLINE_CURVE((1.00061461981704,1.00059701757453,1.))
REPRESENTATION_ITEM('')
);
#296=(
BOUNDED_CURVE()
B_SPLINE_CURVE(2,(#98265,#98266,#98267),.UNSPECIFIED.,.F.,.F.)
B_SPLINE_CURVE_WITH_KNOTS((3,3),(0.,0.060325206882409),.UNSPECIFIED.)
CURVE()
GEOMETRIC_REPRESENTATION_ITEM()
RATIONAL_B_SPLINE_CURVE((1.,1.00059701758008,1.00061461982276))
REPRESENTATION_ITEM('')
);
#297=(
BOUNDED_CURVE()
B_SPLINE_CURVE(2,(#98269,#98270,#98271),.UNSPECIFIED.,.F.,.F.)
B_SPLINE_CURVE_WITH_KNOTS((3,3),(0.0639904841458431,0.124315691028302),
 .UNSPECIFIED.)
CURVE()
GEOMETRIC_REPRESENTATION_ITEM()
RATIONAL_B_SPLINE_CURVE((1.00061461982011,1.0005970175775,1.))
REPRESENTATION_ITEM('')
);
#298=(
BOUNDED_CURVE()
B_SPLINE_CURVE(2,(#98275,#98276,#98277),.UNSPECIFIED.,.F.,.F.)
B_SPLINE_CURVE_WITH_KNOTS((3,3),(0.,0.0603252068824613),.UNSPECIFIED.)
CURVE()
GEOMETRIC_REPRESENTATION_ITEM()
RATIONAL_B_SPLINE_CURVE((1.,1.00059701757306,1.00061461981553))
REPRESENTATION_ITEM('')
);
#299=(
BOUNDED_CURVE()
B_SPLINE_CURVE(2,(#98279,#98280,#98281),.UNSPECIFIED.,.F.,.F.)
B_SPLINE_CURVE_WITH_KNOTS((3,3),(0.0639904841458487,0.124315691028303),
 .UNSPECIFIED.)
CURVE()
GEOMETRIC_REPRESENTATION_ITEM()
RATIONAL_B_SPLINE_CURVE((1.00061461981873,1.00059701757616,1.))
REPRESENTATION_ITEM('')
);
#300=(
BOUNDED_CURVE()
B_SPLINE_CURVE(2,(#98285,#98286,#98287),.UNSPECIFIED.,.F.,.F.)
B_SPLINE_CURVE_WITH_KNOTS((3,3),(0.,0.0603252068824276),.UNSPECIFIED.)
CURVE()
GEOMETRIC_REPRESENTATION_ITEM()
RATIONAL_B_SPLINE_CURVE((1.,1.00059701757807,1.00061461982069))
REPRESENTATION_ITEM('')
);
#301=(
BOUNDED_CURVE()
B_SPLINE_CURVE(2,(#98289,#98290,#98291),.UNSPECIFIED.,.F.,.F.)
B_SPLINE_CURVE_WITH_KNOTS((3,3),(0.0639904841458727,0.124315691028301),
 .UNSPECIFIED.)
CURVE()
GEOMETRIC_REPRESENTATION_ITEM()
RATIONAL_B_SPLINE_CURVE((1.00061461981734,1.00059701757482,1.))
REPRESENTATION_ITEM('')
);
#302=(
BOUNDED_CURVE()
B_SPLINE_CURVE(2,(#98295,#98296,#98297),.UNSPECIFIED.,.F.,.F.)
B_SPLINE_CURVE_WITH_KNOTS((3,3),(0.,0.0603252068823914),.UNSPECIFIED.)
CURVE()
GEOMETRIC_REPRESENTATION_ITEM()
RATIONAL_B_SPLINE_CURVE((1.,1.00059701757592,1.00061461981848))
REPRESENTATION_ITEM('')
);
#303=(
BOUNDED_CURVE()
B_SPLINE_CURVE(2,(#98299,#98300,#98301),.UNSPECIFIED.,.F.,.F.)
B_SPLINE_CURVE_WITH_KNOTS((3,3),(0.063990484145862,0.124315691028302),
 .UNSPECIFIED.)
CURVE()
GEOMETRIC_REPRESENTATION_ITEM()
RATIONAL_B_SPLINE_CURVE((1.00061461982072,1.0005970175781,1.))
REPRESENTATION_ITEM('')
);
#304=(
BOUNDED_CURVE()
B_SPLINE_CURVE(2,(#98305,#98306,#98307),.UNSPECIFIED.,.F.,.F.)
B_SPLINE_CURVE_WITH_KNOTS((3,3),(0.,0.0603252068824525),.UNSPECIFIED.)
CURVE()
GEOMETRIC_REPRESENTATION_ITEM()
RATIONAL_B_SPLINE_CURVE((1.,1.00059701757595,1.00061461981851))
REPRESENTATION_ITEM('')
);
#305=(
BOUNDED_CURVE()
B_SPLINE_CURVE(2,(#98309,#98310,#98311),.UNSPECIFIED.,.F.,.F.)
B_SPLINE_CURVE_WITH_KNOTS((3,3),(0.0639904841458752,0.124315691028301),
 .UNSPECIFIED.)
CURVE()
GEOMETRIC_REPRESENTATION_ITEM()
RATIONAL_B_SPLINE_CURVE((1.00061461981711,1.0005970175746,1.))
REPRESENTATION_ITEM('')
);
#306=(
BOUNDED_CURVE()
B_SPLINE_CURVE(2,(#98315,#98316,#98317),.UNSPECIFIED.,.F.,.F.)
B_SPLINE_CURVE_WITH_KNOTS((3,3),(0.,0.0603252068824554),.UNSPECIFIED.)
CURVE()
GEOMETRIC_REPRESENTATION_ITEM()
RATIONAL_B_SPLINE_CURVE((1.,1.00059701757617,1.00061461981873))
REPRESENTATION_ITEM('')
);
#307=(
BOUNDED_CURVE()
B_SPLINE_CURVE(2,(#98319,#98320,#98321),.UNSPECIFIED.,.F.,.F.)
B_SPLINE_CURVE_WITH_KNOTS((3,3),(0.0639904841458758,0.124315691028301),
 .UNSPECIFIED.)
CURVE()
GEOMETRIC_REPRESENTATION_ITEM()
RATIONAL_B_SPLINE_CURVE((1.00061461982041,1.0005970175778,1.))
REPRESENTATION_ITEM('')
);
#308=(
BOUNDED_CURVE()
B_SPLINE_CURVE(2,(#98325,#98326,#98327),.UNSPECIFIED.,.F.,.F.)
B_SPLINE_CURVE_WITH_KNOTS((3,3),(0.,0.0603252068824492),.UNSPECIFIED.)
CURVE()
GEOMETRIC_REPRESENTATION_ITEM()
RATIONAL_B_SPLINE_CURVE((1.,1.00059701757446,1.00061461981697))
REPRESENTATION_ITEM('')
);
#309=(
BOUNDED_CURVE()
B_SPLINE_CURVE(2,(#98329,#98330,#98331),.UNSPECIFIED.,.F.,.F.)
B_SPLINE_CURVE_WITH_KNOTS((3,3),(0.0639904841458399,0.124315691028302),
 .UNSPECIFIED.)
CURVE()
GEOMETRIC_REPRESENTATION_ITEM()
RATIONAL_B_SPLINE_CURVE((1.00061461981953,1.00059701757694,1.))
REPRESENTATION_ITEM('')
);
#310=(
BOUNDED_CURVE()
B_SPLINE_CURVE(2,(#98335,#98336,#98337),.UNSPECIFIED.,.F.,.F.)
B_SPLINE_CURVE_WITH_KNOTS((3,3),(0.,0.060325206882422),.UNSPECIFIED.)
CURVE()
GEOMETRIC_REPRESENTATION_ITEM()
RATIONAL_B_SPLINE_CURVE((1.,1.00059701757302,1.00061461981549))
REPRESENTATION_ITEM('')
);
#311=(
BOUNDED_CURVE()
B_SPLINE_CURVE(2,(#98339,#98340,#98341),.UNSPECIFIED.,.F.,.F.)
B_SPLINE_CURVE_WITH_KNOTS((3,3),(0.0639904841458821,0.124315691028301),
 .UNSPECIFIED.)
CURVE()
GEOMETRIC_REPRESENTATION_ITEM()
RATIONAL_B_SPLINE_CURVE((1.00061461982,1.0005970175774,1.))
REPRESENTATION_ITEM('')
);
#312=(
BOUNDED_CURVE()
B_SPLINE_CURVE(2,(#98345,#98346,#98347),.UNSPECIFIED.,.F.,.F.)
B_SPLINE_CURVE_WITH_KNOTS((3,3),(0.,0.060325206882426),.UNSPECIFIED.)
CURVE()
GEOMETRIC_REPRESENTATION_ITEM()
RATIONAL_B_SPLINE_CURVE((1.,1.0005970175762,1.00061461981876))
REPRESENTATION_ITEM('')
);
#313=(
BOUNDED_CURVE()
B_SPLINE_CURVE(2,(#98349,#98350,#98351),.UNSPECIFIED.,.F.,.F.)
B_SPLINE_CURVE_WITH_KNOTS((3,3),(0.0639904841458618,0.124315691028301),
 .UNSPECIFIED.)
CURVE()
GEOMETRIC_REPRESENTATION_ITEM()
RATIONAL_B_SPLINE_CURVE((1.00061461981851,1.00059701757596,1.))
REPRESENTATION_ITEM('')
);
#314=(
BOUNDED_CURVE()
B_SPLINE_CURVE(2,(#98355,#98356,#98357),.UNSPECIFIED.,.F.,.F.)
B_SPLINE_CURVE_WITH_KNOTS((3,3),(0.,0.060325206882439),.UNSPECIFIED.)
CURVE()
GEOMETRIC_REPRESENTATION_ITEM()
RATIONAL_B_SPLINE_CURVE((1.,1.000597017576,1.00061461981855))
REPRESENTATION_ITEM('')
);
#315=(
BOUNDED_CURVE()
B_SPLINE_CURVE(2,(#98359,#98360,#98361),.UNSPECIFIED.,.F.,.F.)
B_SPLINE_CURVE_WITH_KNOTS((3,3),(0.0639904841458451,0.124315691028302),
 .UNSPECIFIED.)
CURVE()
GEOMETRIC_REPRESENTATION_ITEM()
RATIONAL_B_SPLINE_CURVE((1.00061461981588,1.0005970175734,1.))
REPRESENTATION_ITEM('')
);
#316=(
BOUNDED_CURVE()
B_SPLINE_CURVE(2,(#98365,#98366,#98367),.UNSPECIFIED.,.F.,.F.)
B_SPLINE_CURVE_WITH_KNOTS((3,3),(0.,0.0603252068824284),.UNSPECIFIED.)
CURVE()
GEOMETRIC_REPRESENTATION_ITEM()
RATIONAL_B_SPLINE_CURVE((1.,1.0005970175755,1.00061461981804))
REPRESENTATION_ITEM('')
);
#317=(
BOUNDED_CURVE()
B_SPLINE_CURVE(2,(#98369,#98370,#98371),.UNSPECIFIED.,.F.,.F.)
B_SPLINE_CURVE_WITH_KNOTS((3,3),(0.063990484145897,0.124315691028301),
 .UNSPECIFIED.)
CURVE()
GEOMETRIC_REPRESENTATION_ITEM()
RATIONAL_B_SPLINE_CURVE((1.00061461982066,1.00059701757804,1.))
REPRESENTATION_ITEM('')
);
#318=(
BOUNDED_CURVE()
B_SPLINE_CURVE(2,(#98375,#98376,#98377),.UNSPECIFIED.,.F.,.F.)
B_SPLINE_CURVE_WITH_KNOTS((3,3),(0.,0.0603252068824418),.UNSPECIFIED.)
CURVE()
GEOMETRIC_REPRESENTATION_ITEM()
RATIONAL_B_SPLINE_CURVE((1.,1.00059701757692,1.00061461981951))
REPRESENTATION_ITEM('')
);
#319=(
BOUNDED_CURVE()
B_SPLINE_CURVE(2,(#98379,#98380,#98381),.UNSPECIFIED.,.F.,.F.)
B_SPLINE_CURVE_WITH_KNOTS((3,3),(0.063990484145828,0.124315691028302),
 .UNSPECIFIED.)
CURVE()
GEOMETRIC_REPRESENTATION_ITEM()
RATIONAL_B_SPLINE_CURVE((1.00061461982019,1.00059701757759,1.))
REPRESENTATION_ITEM('')
);
#320=(
BOUNDED_CURVE()
B_SPLINE_CURVE(2,(#98385,#98386,#98387),.UNSPECIFIED.,.F.,.F.)
B_SPLINE_CURVE_WITH_KNOTS((3,3),(0.,0.0603252068824602),.UNSPECIFIED.)
CURVE()
GEOMETRIC_REPRESENTATION_ITEM()
RATIONAL_B_SPLINE_CURVE((1.,1.00059701757713,1.00061461981972))
REPRESENTATION_ITEM('')
);
#321=(
BOUNDED_CURVE()
B_SPLINE_CURVE(2,(#98389,#98390,#98391),.UNSPECIFIED.,.F.,.F.)
B_SPLINE_CURVE_WITH_KNOTS((3,3),(0.0639904841458735,0.124315691028303),
 .UNSPECIFIED.)
CURVE()
GEOMETRIC_REPRESENTATION_ITEM()
RATIONAL_B_SPLINE_CURVE((1.00061461982132,1.00059701757868,1.))
REPRESENTATION_ITEM('')
);
#322=(
BOUNDED_CURVE()
B_SPLINE_CURVE(2,(#98395,#98396,#98397),.UNSPECIFIED.,.F.,.F.)
B_SPLINE_CURVE_WITH_KNOTS((3,3),(0.,0.060325206882423),.UNSPECIFIED.)
CURVE()
GEOMETRIC_REPRESENTATION_ITEM()
RATIONAL_B_SPLINE_CURVE((1.,1.00059701757739,1.00061461981999))
REPRESENTATION_ITEM('')
);
#323=(
BOUNDED_CURVE()
B_SPLINE_CURVE(2,(#98399,#98400,#98401),.UNSPECIFIED.,.F.,.F.)
B_SPLINE_CURVE_WITH_KNOTS((3,3),(0.0639904841458232,0.124315691028303),
 .UNSPECIFIED.)
CURVE()
GEOMETRIC_REPRESENTATION_ITEM()
RATIONAL_B_SPLINE_CURVE((1.00061461981322,1.00059701757082,1.))
REPRESENTATION_ITEM('')
);
#324=(
BOUNDED_CURVE()
B_SPLINE_CURVE(2,(#98405,#98406,#98407),.UNSPECIFIED.,.F.,.F.)
B_SPLINE_CURVE_WITH_KNOTS((3,3),(0.,0.0603252068824245),.UNSPECIFIED.)
CURVE()
GEOMETRIC_REPRESENTATION_ITEM()
RATIONAL_B_SPLINE_CURVE((1.,1.0005970175778,1.00061461982041))
REPRESENTATION_ITEM('')
);
#325=(
BOUNDED_CURVE()
B_SPLINE_CURVE(2,(#98409,#98410,#98411),.UNSPECIFIED.,.F.,.F.)
B_SPLINE_CURVE_WITH_KNOTS((3,3),(0.0639904841458354,0.124315691028301),
 .UNSPECIFIED.)
CURVE()
GEOMETRIC_REPRESENTATION_ITEM()
RATIONAL_B_SPLINE_CURVE((1.00061461981561,1.00059701757313,1.))
REPRESENTATION_ITEM('')
);
#326=(
BOUNDED_CURVE()
B_SPLINE_CURVE(2,(#98415,#98416,#98417),.UNSPECIFIED.,.F.,.F.)
B_SPLINE_CURVE_WITH_KNOTS((3,3),(0.,0.0603252068824727),.UNSPECIFIED.)
CURVE()
GEOMETRIC_REPRESENTATION_ITEM()
RATIONAL_B_SPLINE_CURVE((1.,1.00059701757521,1.00061461981774))
REPRESENTATION_ITEM('')
);
#327=(
BOUNDED_CURVE()
B_SPLINE_CURVE(2,(#98419,#98420,#98421),.UNSPECIFIED.,.F.,.F.)
B_SPLINE_CURVE_WITH_KNOTS((3,3),(0.0639904841458599,0.124315691028302),
 .UNSPECIFIED.)
CURVE()
GEOMETRIC_REPRESENTATION_ITEM()
RATIONAL_B_SPLINE_CURVE((1.00061461981724,1.00059701757472,1.))
REPRESENTATION_ITEM('')
);
#328=(
BOUNDED_CURVE()
B_SPLINE_CURVE(2,(#98425,#98426,#98427),.UNSPECIFIED.,.F.,.F.)
B_SPLINE_CURVE_WITH_KNOTS((3,3),(0.,0.060325206882435),.UNSPECIFIED.)
CURVE()
GEOMETRIC_REPRESENTATION_ITEM()
RATIONAL_B_SPLINE_CURVE((1.,1.000597017572,1.00061461981444))
REPRESENTATION_ITEM('')
);
#329=(
BOUNDED_CURVE()
B_SPLINE_CURVE(2,(#98428,#98429,#98430),.UNSPECIFIED.,.F.,.F.)
B_SPLINE_CURVE_WITH_KNOTS((3,3),(0.0639904841458783,0.124315691028301),
 .UNSPECIFIED.)
CURVE()
GEOMETRIC_REPRESENTATION_ITEM()
RATIONAL_B_SPLINE_CURVE((1.00061461981787,1.00059701757533,1.))
REPRESENTATION_ITEM('')
);
#330=(
BOUNDED_CURVE()
B_SPLINE_CURVE(2,(#98432,#98433,#98434),.UNSPECIFIED.,.F.,.F.)
B_SPLINE_CURVE_WITH_KNOTS((3,3),(0.,0.0603252068824676),.UNSPECIFIED.)
CURVE()
GEOMETRIC_REPRESENTATION_ITEM()
RATIONAL_B_SPLINE_CURVE((1.,1.00059701757413,1.00061461981663))
REPRESENTATION_ITEM('')
);
#331=(
BOUNDED_CURVE()
B_SPLINE_CURVE(2,(#98436,#98437,#98438),.UNSPECIFIED.,.F.,.F.)
B_SPLINE_CURVE_WITH_KNOTS((3,3),(0.0639904841458132,0.124315691028303),
 .UNSPECIFIED.)
CURVE()
GEOMETRIC_REPRESENTATION_ITEM()
RATIONAL_B_SPLINE_CURVE((1.00061461981527,1.0005970175728,1.))
REPRESENTATION_ITEM('')
);
#332=(
BOUNDED_CURVE()
B_SPLINE_CURVE(2,(#98442,#98443,#98444),.UNSPECIFIED.,.F.,.F.)
B_SPLINE_CURVE_WITH_KNOTS((3,3),(0.,0.0603252068824029),.UNSPECIFIED.)
CURVE()
GEOMETRIC_REPRESENTATION_ITEM()
RATIONAL_B_SPLINE_CURVE((1.,1.00059701757378,1.00061461981628))
REPRESENTATION_ITEM('')
);
#333=(
BOUNDED_CURVE()
B_SPLINE_CURVE(2,(#98446,#98447,#98448),.UNSPECIFIED.,.F.,.F.)
B_SPLINE_CURVE_WITH_KNOTS((3,3),(0.0639904841458425,0.124315691028302),
 .UNSPECIFIED.)
CURVE()
GEOMETRIC_REPRESENTATION_ITEM()
RATIONAL_B_SPLINE_CURVE((1.0006146198229,1.00059701758022,1.))
REPRESENTATION_ITEM('')
);
#334=(
BOUNDED_CURVE()
B_SPLINE_CURVE(2,(#98452,#98453,#98454),.UNSPECIFIED.,.F.,.F.)
B_SPLINE_CURVE_WITH_KNOTS((3,3),(0.,0.0603252068824536),.UNSPECIFIED.)
CURVE()
GEOMETRIC_REPRESENTATION_ITEM()
RATIONAL_B_SPLINE_CURVE((1.,1.00059701757467,1.00061461981719))
REPRESENTATION_ITEM('')
);
#335=(
BOUNDED_CURVE()
B_SPLINE_CURVE(2,(#98456,#98457,#98458),.UNSPECIFIED.,.F.,.F.)
B_SPLINE_CURVE_WITH_KNOTS((3,3),(0.0639904841458365,0.124315691028303),
 .UNSPECIFIED.)
CURVE()
GEOMETRIC_REPRESENTATION_ITEM()
RATIONAL_B_SPLINE_CURVE((1.00061461981477,1.00059701757232,1.))
REPRESENTATION_ITEM('')
);
#336=(
BOUNDED_CURVE()
B_SPLINE_CURVE(2,(#98462,#98463,#98464),.UNSPECIFIED.,.F.,.F.)
B_SPLINE_CURVE_WITH_KNOTS((3,3),(0.,0.0603252068824354),.UNSPECIFIED.)
CURVE()
GEOMETRIC_REPRESENTATION_ITEM()
RATIONAL_B_SPLINE_CURVE((1.,1.00059701758002,1.0006146198227))
REPRESENTATION_ITEM('')
);
#337=(
BOUNDED_CURVE()
B_SPLINE_CURVE(2,(#98466,#98467,#98468),.UNSPECIFIED.,.F.,.F.)
B_SPLINE_CURVE_WITH_KNOTS((3,3),(0.0639904841458278,0.124315691028302),
 .UNSPECIFIED.)
CURVE()
GEOMETRIC_REPRESENTATION_ITEM()
RATIONAL_B_SPLINE_CURVE((1.00061461981225,1.00059701756987,1.))
REPRESENTATION_ITEM('')
);
#338=(
BOUNDED_CURVE()
B_SPLINE_CURVE(2,(#98472,#98473,#98474),.UNSPECIFIED.,.F.,.F.)
B_SPLINE_CURVE_WITH_KNOTS((3,3),(0.,0.0603252068824639),.UNSPECIFIED.)
CURVE()
GEOMETRIC_REPRESENTATION_ITEM()
RATIONAL_B_SPLINE_CURVE((1.,1.000597017572,1.00061461981444))
REPRESENTATION_ITEM('')
);
#339=(
BOUNDED_CURVE()
B_SPLINE_CURVE(2,(#98476,#98477,#98478),.UNSPECIFIED.,.F.,.F.)
B_SPLINE_CURVE_WITH_KNOTS((3,3),(0.0639904841458256,0.124315691028302),
 .UNSPECIFIED.)
CURVE()
GEOMETRIC_REPRESENTATION_ITEM()
RATIONAL_B_SPLINE_CURVE((1.00061461981674,1.00059701757424,1.))
REPRESENTATION_ITEM('')
);
#340=(
BOUNDED_CURVE()
B_SPLINE_CURVE(2,(#98482,#98483,#98484),.UNSPECIFIED.,.F.,.F.)
B_SPLINE_CURVE_WITH_KNOTS((3,3),(0.,0.0603252068824755),.UNSPECIFIED.)
CURVE()
GEOMETRIC_REPRESENTATION_ITEM()
RATIONAL_B_SPLINE_CURVE((1.,1.00059701757238,1.00061461981483))
REPRESENTATION_ITEM('')
);
#341=(
BOUNDED_CURVE()
B_SPLINE_CURVE(2,(#98486,#98487,#98488),.UNSPECIFIED.,.F.,.F.)
B_SPLINE_CURVE_WITH_KNOTS((3,3),(0.0639904841458611,0.124315691028301),
 .UNSPECIFIED.)
CURVE()
GEOMETRIC_REPRESENTATION_ITEM()
RATIONAL_B_SPLINE_CURVE((1.00061461981833,1.00059701757578,1.))
REPRESENTATION_ITEM('')
);
#342=(
BOUNDED_CURVE()
B_SPLINE_CURVE(2,(#98492,#98493,#98494),.UNSPECIFIED.,.F.,.F.)
B_SPLINE_CURVE_WITH_KNOTS((3,3),(0.,0.0603252068824602),.UNSPECIFIED.)
CURVE()
GEOMETRIC_REPRESENTATION_ITEM()
RATIONAL_B_SPLINE_CURVE((1.,1.00059701757416,1.00061461981667))
REPRESENTATION_ITEM('')
);
#343=(
BOUNDED_CURVE()
B_SPLINE_CURVE(2,(#98496,#98497,#98498),.UNSPECIFIED.,.F.,.F.)
B_SPLINE_CURVE_WITH_KNOTS((3,3),(0.063990484145903,0.124315691028301),
 .UNSPECIFIED.)
CURVE()
GEOMETRIC_REPRESENTATION_ITEM()
RATIONAL_B_SPLINE_CURVE((1.00061461981856,1.00059701757601,1.))
REPRESENTATION_ITEM('')
);
#344=(
BOUNDED_CURVE()
B_SPLINE_CURVE(2,(#98502,#98503,#98504),.UNSPECIFIED.,.F.,.F.)
B_SPLINE_CURVE_WITH_KNOTS((3,3),(0.,0.060325206882481),.UNSPECIFIED.)
CURVE()
GEOMETRIC_REPRESENTATION_ITEM()
RATIONAL_B_SPLINE_CURVE((1.,1.00059701757576,1.00061461981831))
REPRESENTATION_ITEM('')
);
#345=(
BOUNDED_CURVE()
B_SPLINE_CURVE(2,(#98506,#98507,#98508),.UNSPECIFIED.,.F.,.F.)
B_SPLINE_CURVE_WITH_KNOTS((3,3),(0.0639904841458541,0.124315691028302),
 .UNSPECIFIED.)
CURVE()
GEOMETRIC_REPRESENTATION_ITEM()
RATIONAL_B_SPLINE_CURVE((1.00061461982049,1.00059701757788,1.))
REPRESENTATION_ITEM('')
);
#346=(
BOUNDED_CURVE()
B_SPLINE_CURVE(2,(#98512,#98513,#98514),.UNSPECIFIED.,.F.,.F.)
B_SPLINE_CURVE_WITH_KNOTS((3,3),(0.,0.0603252068824261),.UNSPECIFIED.)
CURVE()
GEOMETRIC_REPRESENTATION_ITEM()
RATIONAL_B_SPLINE_CURVE((1.,1.00059701757482,1.00061461981734))
REPRESENTATION_ITEM('')
);
#347=(
BOUNDED_CURVE()
B_SPLINE_CURVE(2,(#98516,#98517,#98518),.UNSPECIFIED.,.F.,.F.)
B_SPLINE_CURVE_WITH_KNOTS((3,3),(0.0639904841458672,0.124315691028302),
 .UNSPECIFIED.)
CURVE()
GEOMETRIC_REPRESENTATION_ITEM()
RATIONAL_B_SPLINE_CURVE((1.00061461981919,1.00059701757661,1.))
REPRESENTATION_ITEM('')
);
#348=(
BOUNDED_CURVE()
B_SPLINE_CURVE(2,(#98522,#98523,#98524),.UNSPECIFIED.,.F.,.F.)
B_SPLINE_CURVE_WITH_KNOTS((3,3),(0.,0.0603252068824262),.UNSPECIFIED.)
CURVE()
GEOMETRIC_REPRESENTATION_ITEM()
RATIONAL_B_SPLINE_CURVE((1.,1.00059701757468,1.0006146198172))
REPRESENTATION_ITEM('')
);
#349=(
BOUNDED_CURVE()
B_SPLINE_CURVE(2,(#98526,#98527,#98528),.UNSPECIFIED.,.F.,.F.)
B_SPLINE_CURVE_WITH_KNOTS((3,3),(0.0639904841458652,0.124315691028301),
 .UNSPECIFIED.)
CURVE()
GEOMETRIC_REPRESENTATION_ITEM()
RATIONAL_B_SPLINE_CURVE((1.00061461982038,1.00059701757777,1.))
REPRESENTATION_ITEM('')
);
#350=(
BOUNDED_CURVE()
B_SPLINE_CURVE(2,(#98532,#98533,#98534),.UNSPECIFIED.,.F.,.F.)
B_SPLINE_CURVE_WITH_KNOTS((3,3),(0.,0.0603252068824703),.UNSPECIFIED.)
CURVE()
GEOMETRIC_REPRESENTATION_ITEM()
RATIONAL_B_SPLINE_CURVE((1.,1.00059701757448,1.00061461981699))
REPRESENTATION_ITEM('')
);
#351=(
BOUNDED_CURVE()
B_SPLINE_CURVE(2,(#98536,#98537,#98538),.UNSPECIFIED.,.F.,.F.)
B_SPLINE_CURVE_WITH_KNOTS((3,3),(0.0639904841458294,0.124315691028302),
 .UNSPECIFIED.)
CURVE()
GEOMETRIC_REPRESENTATION_ITEM()
RATIONAL_B_SPLINE_CURVE((1.00061461981863,1.00059701757607,1.))
REPRESENTATION_ITEM('')
);
#352=(
BOUNDED_CURVE()
B_SPLINE_CURVE(2,(#98542,#98543,#98544),.UNSPECIFIED.,.F.,.F.)
B_SPLINE_CURVE_WITH_KNOTS((3,3),(0.,0.0603252068824115),.UNSPECIFIED.)
CURVE()
GEOMETRIC_REPRESENTATION_ITEM()
RATIONAL_B_SPLINE_CURVE((1.,1.00059701757804,1.00061461982066))
REPRESENTATION_ITEM('')
);
#353=(
BOUNDED_CURVE()
B_SPLINE_CURVE(2,(#98546,#98547,#98548),.UNSPECIFIED.,.F.,.F.)
B_SPLINE_CURVE_WITH_KNOTS((3,3),(0.0639904841458776,0.124315691028301),
 .UNSPECIFIED.)
CURVE()
GEOMETRIC_REPRESENTATION_ITEM()
RATIONAL_B_SPLINE_CURVE((1.00061461981868,1.00059701757612,1.))
REPRESENTATION_ITEM('')
);
#354=(
BOUNDED_CURVE()
B_SPLINE_CURVE(2,(#98552,#98553,#98554),.UNSPECIFIED.,.F.,.F.)
B_SPLINE_CURVE_WITH_KNOTS((3,3),(0.,0.0603252068824542),.UNSPECIFIED.)
CURVE()
GEOMETRIC_REPRESENTATION_ITEM()
RATIONAL_B_SPLINE_CURVE((1.,1.00059701757636,1.00061461981893))
REPRESENTATION_ITEM('')
);
#355=(
BOUNDED_CURVE()
B_SPLINE_CURVE(2,(#98556,#98557,#98558),.UNSPECIFIED.,.F.,.F.)
B_SPLINE_CURVE_WITH_KNOTS((3,3),(0.0639904841459132,0.124315691028299),
 .UNSPECIFIED.)
CURVE()
GEOMETRIC_REPRESENTATION_ITEM()
RATIONAL_B_SPLINE_CURVE((1.00061461981658,1.00059701757408,1.))
REPRESENTATION_ITEM('')
);
#356=(
BOUNDED_CURVE()
B_SPLINE_CURVE(2,(#98562,#98563,#98564),.UNSPECIFIED.,.F.,.F.)
B_SPLINE_CURVE_WITH_KNOTS((3,3),(0.,0.060325206882438),.UNSPECIFIED.)
CURVE()
GEOMETRIC_REPRESENTATION_ITEM()
RATIONAL_B_SPLINE_CURVE((1.,1.00059701757669,1.00061461981927))
REPRESENTATION_ITEM('')
);
#357=(
BOUNDED_CURVE()
B_SPLINE_CURVE(2,(#98566,#98567,#98568),.UNSPECIFIED.,.F.,.F.)
B_SPLINE_CURVE_WITH_KNOTS((3,3),(0.0639904841458312,0.124315691028303),
 .UNSPECIFIED.)
CURVE()
GEOMETRIC_REPRESENTATION_ITEM()
RATIONAL_B_SPLINE_CURVE((1.00061461982088,1.00059701757825,1.))
REPRESENTATION_ITEM('')
);
#358=(
BOUNDED_CURVE()
B_SPLINE_CURVE(2,(#98572,#98573,#98574),.UNSPECIFIED.,.F.,.F.)
B_SPLINE_CURVE_WITH_KNOTS((3,3),(0.,0.0603252068824436),.UNSPECIFIED.)
CURVE()
GEOMETRIC_REPRESENTATION_ITEM()
RATIONAL_B_SPLINE_CURVE((1.,1.00059701757611,1.00061461981868))
REPRESENTATION_ITEM('')
);
#359=(
BOUNDED_CURVE()
B_SPLINE_CURVE(2,(#98576,#98577,#98578),.UNSPECIFIED.,.F.,.F.)
B_SPLINE_CURVE_WITH_KNOTS((3,3),(0.0639904841458248,0.124315691028303),
 .UNSPECIFIED.)
CURVE()
GEOMETRIC_REPRESENTATION_ITEM()
RATIONAL_B_SPLINE_CURVE((1.00061461981152,1.00059701756916,1.))
REPRESENTATION_ITEM('')
);
#360=(
BOUNDED_CURVE()
B_SPLINE_CURVE(2,(#98582,#98583,#98584),.UNSPECIFIED.,.F.,.F.)
B_SPLINE_CURVE_WITH_KNOTS((3,3),(0.,0.060325206882417),.UNSPECIFIED.)
CURVE()
GEOMETRIC_REPRESENTATION_ITEM()
RATIONAL_B_SPLINE_CURVE((1.,1.00059701758071,1.0006146198234))
REPRESENTATION_ITEM('')
);
#361=(
BOUNDED_CURVE()
B_SPLINE_CURVE(2,(#98586,#98587,#98588),.UNSPECIFIED.,.F.,.F.)
B_SPLINE_CURVE_WITH_KNOTS((3,3),(0.063990484145854,0.124315691028302),
 .UNSPECIFIED.)
CURVE()
GEOMETRIC_REPRESENTATION_ITEM()
RATIONAL_B_SPLINE_CURVE((1.00061461982008,1.00059701757748,1.))
REPRESENTATION_ITEM('')
);
#362=(
BOUNDED_CURVE()
B_SPLINE_CURVE(2,(#98592,#98593,#98594),.UNSPECIFIED.,.F.,.F.)
B_SPLINE_CURVE_WITH_KNOTS((3,3),(0.,0.0603252068824378),.UNSPECIFIED.)
CURVE()
GEOMETRIC_REPRESENTATION_ITEM()
RATIONAL_B_SPLINE_CURVE((1.,1.00059701757204,1.00061461981449))
REPRESENTATION_ITEM('')
);
#363=(
BOUNDED_CURVE()
B_SPLINE_CURVE(2,(#98596,#98597,#98598),.UNSPECIFIED.,.F.,.F.)
B_SPLINE_CURVE_WITH_KNOTS((3,3),(0.0639904841458379,0.124315691028302),
 .UNSPECIFIED.)
CURVE()
GEOMETRIC_REPRESENTATION_ITEM()
RATIONAL_B_SPLINE_CURVE((1.00061461981444,1.000597017572,1.))
REPRESENTATION_ITEM('')
);
#364=(
BOUNDED_CURVE()
B_SPLINE_CURVE(2,(#98602,#98603,#98604),.UNSPECIFIED.,.F.,.F.)
B_SPLINE_CURVE_WITH_KNOTS((3,3),(0.,0.0603252068824703),.UNSPECIFIED.)
CURVE()
GEOMETRIC_REPRESENTATION_ITEM()
RATIONAL_B_SPLINE_CURVE((1.,1.00059701757202,1.00061461981446))
REPRESENTATION_ITEM('')
);
#365=(
BOUNDED_CURVE()
B_SPLINE_CURVE(2,(#98606,#98607,#98608),.UNSPECIFIED.,.F.,.F.)
B_SPLINE_CURVE_WITH_KNOTS((3,3),(0.0639904841458564,0.124315691028301),
 .UNSPECIFIED.)
CURVE()
GEOMETRIC_REPRESENTATION_ITEM()
RATIONAL_B_SPLINE_CURVE((1.00061461982062,1.000597017578,1.))
REPRESENTATION_ITEM('')
);
#366=(
BOUNDED_CURVE()
B_SPLINE_CURVE(2,(#98612,#98613,#98614),.UNSPECIFIED.,.F.,.F.)
B_SPLINE_CURVE_WITH_KNOTS((3,3),(0.,0.0603252068824437),.UNSPECIFIED.)
CURVE()
GEOMETRIC_REPRESENTATION_ITEM()
RATIONAL_B_SPLINE_CURVE((1.,1.00059701757562,1.00061461981817))
REPRESENTATION_ITEM('')
);
#367=(
BOUNDED_CURVE()
B_SPLINE_CURVE(2,(#98616,#98617,#98618),.UNSPECIFIED.,.F.,.F.)
B_SPLINE_CURVE_WITH_KNOTS((3,3),(0.0639904841458463,0.124315691028302),
 .UNSPECIFIED.)
CURVE()
GEOMETRIC_REPRESENTATION_ITEM()
RATIONAL_B_SPLINE_CURVE((1.00061461981433,1.0005970175719,1.))
REPRESENTATION_ITEM('')
);
#368=(
BOUNDED_CURVE()
B_SPLINE_CURVE(2,(#98622,#98623,#98624),.UNSPECIFIED.,.F.,.F.)
B_SPLINE_CURVE_WITH_KNOTS((3,3),(0.,0.0603252068824302),.UNSPECIFIED.)
CURVE()
GEOMETRIC_REPRESENTATION_ITEM()
RATIONAL_B_SPLINE_CURVE((1.,1.00059701757328,1.00061461981576))
REPRESENTATION_ITEM('')
);
#369=(
BOUNDED_CURVE()
B_SPLINE_CURVE(2,(#98626,#98627,#98628),.UNSPECIFIED.,.F.,.F.)
B_SPLINE_CURVE_WITH_KNOTS((3,3),(0.06399048414589,0.1243156910283),
 .UNSPECIFIED.)
CURVE()
GEOMETRIC_REPRESENTATION_ITEM()
RATIONAL_B_SPLINE_CURVE((1.00061461981725,1.00059701757473,1.))
REPRESENTATION_ITEM('')
);
#370=(
BOUNDED_CURVE()
B_SPLINE_CURVE(2,(#98631,#98632,#98633),.UNSPECIFIED.,.F.,.F.)
B_SPLINE_CURVE_WITH_KNOTS((3,3),(0.,0.0603252068825018),.UNSPECIFIED.)
CURVE()
GEOMETRIC_REPRESENTATION_ITEM()
RATIONAL_B_SPLINE_CURVE((1.,1.00059701757198,1.00061461981442))
REPRESENTATION_ITEM('')
);
#520=SHAPE_REPRESENTATION_RELATIONSHIP('SRR','None',#114057,#538);
#538=ADVANCED_BREP_SHAPE_REPRESENTATION('',(#574),#113971);
#556=STYLED_ITEM('',(#114324),#574);
#574=MANIFOLD_SOLID_BREP('Knurled Adjustment Knob D20',#60397);
#656=CYLINDRICAL_SURFACE('',#62142,1.54999999999999);
#657=CYLINDRICAL_SURFACE('',#62189,10.);
#658=CYLINDRICAL_SURFACE('',#62191,10.);
#659=CYLINDRICAL_SURFACE('',#62195,10.);
#660=CYLINDRICAL_SURFACE('',#62240,10.);
#661=CYLINDRICAL_SURFACE('',#62241,10.);
#662=CYLINDRICAL_SURFACE('',#62244,10.);
#663=CYLINDRICAL_SURFACE('',#62249,10.);
#664=CYLINDRICAL_SURFACE('',#62250,10.);
#665=CYLINDRICAL_SURFACE('',#62253,10.);
#666=CYLINDRICAL_SURFACE('',#62258,10.);
#667=CYLINDRICAL_SURFACE('',#62259,10.);
#668=CYLINDRICAL_SURFACE('',#62262,10.);
#669=CYLINDRICAL_SURFACE('',#62267,10.);
#670=CYLINDRICAL_SURFACE('',#62268,10.);
#671=CYLINDRICAL_SURFACE('',#62271,10.);
#672=CYLINDRICAL_SURFACE('',#62276,10.);
#673=CYLINDRICAL_SURFACE('',#62277,10.);
#674=CYLINDRICAL_SURFACE('',#62280,10.);
#675=CYLINDRICAL_SURFACE('',#62285,10.);
#676=CYLINDRICAL_SURFACE('',#62286,10.);
#677=CYLINDRICAL_SURFACE('',#62289,10.);
#678=CYLINDRICAL_SURFACE('',#62294,10.);
#679=CYLINDRICAL_SURFACE('',#62295,10.);
#680=CYLINDRICAL_SURFACE('',#62298,10.);
#681=CYLINDRICAL_SURFACE('',#62303,10.);
#682=CYLINDRICAL_SURFACE('',#62304,10.);
#683=CYLINDRICAL_SURFACE('',#62307,10.);
#684=CYLINDRICAL_SURFACE('',#62312,10.);
#685=CYLINDRICAL_SURFACE('',#62313,10.);
#686=CYLINDRICAL_SURFACE('',#62316,10.);
#687=CYLINDRICAL_SURFACE('',#62321,10.);
#688=CYLINDRICAL_SURFACE('',#62322,10.);
#689=CYLINDRICAL_SURFACE('',#62325,10.);
#690=CYLINDRICAL_SURFACE('',#62330,10.);
#691=CYLINDRICAL_SURFACE('',#62331,10.);
#692=CYLINDRICAL_SURFACE('',#62334,10.);
#693=CYLINDRICAL_SURFACE('',#62339,10.);
#694=CYLINDRICAL_SURFACE('',#62340,10.);
#695=CYLINDRICAL_SURFACE('',#62343,10.);
#696=CYLINDRICAL_SURFACE('',#62355,4.);
#697=CYLINDRICAL_SURFACE('',#62361,6.);
#698=CYLINDRICAL_SURFACE('',#62366,10.);
#699=CYLINDRICAL_SURFACE('',#62374,2.51000000000001);
#914=CONICAL_SURFACE('',#62147,9.60000000000001,0.785398163397448);
#915=CONICAL_SURFACE('',#62197,9.60000000000001,0.785398163397448);
#916=CONICAL_SURFACE('',#62348,2.66000000000002,0.785398163397448);
#917=CONICAL_SURFACE('',#62353,3.85000000000002,0.785398163397448);
#918=CONICAL_SURFACE('',#62357,4.20000000000002,0.785398163397459);
#919=CONICAL_SURFACE('',#62363,6.20000000000001,0.785398163397459);
#920=CONICAL_SURFACE('',#62369,7.19999999999999,0.785398163397448);
#921=CONICAL_SURFACE('',#62372,1.25500000000001,1.0321363555003);
#1137=CIRCLE('',#62140,1.54999999999999);
#1138=CIRCLE('',#62141,1.54999999999999);
#1139=CIRCLE('',#62143,1.54999999999999);
#1140=CIRCLE('',#62148,10.);
#1141=CIRCLE('',#62149,10.);
#1142=CIRCLE('',#62150,10.);
#1143=CIRCLE('',#62151,10.);
#1144=CIRCLE('',#62152,10.);
#1145=CIRCLE('',#62153,10.);
#1146=CIRCLE('',#62154,10.);
#1147=CIRCLE('',#62155,10.);
#1148=CIRCLE('',#62156,10.);
#1149=CIRCLE('',#62157,10.);
#1150=CIRCLE('',#62158,10.);
#1151=CIRCLE('',#62159,10.);
#1152=CIRCLE('',#62160,10.);
#1153=CIRCLE('',#62161,10.);
#1154=CIRCLE('',#62162,10.);
#1155=CIRCLE('',#62163,10.);
#1156=CIRCLE('',#62164,10.);
#1157=CIRCLE('',#62165,10.);
#1158=CIRCLE('',#62166,10.);
#1159=CIRCLE('',#62167,9.2);
#1160=CIRCLE('',#62168,10.);
#1161=CIRCLE('',#62169,10.);
#1162=CIRCLE('',#62170,10.);
#1163=CIRCLE('',#62171,10.);
#1164=CIRCLE('',#62172,10.);
#1165=CIRCLE('',#62173,10.);
#1166=CIRCLE('',#62174,10.);
#1167=CIRCLE('',#62175,10.);
#1168=CIRCLE('',#62176,10.);
#1169=CIRCLE('',#62177,10.);
#1170=CIRCLE('',#62178,10.);
#1171=CIRCLE('',#62179,10.);
#1172=CIRCLE('',#62180,10.);
#1173=CIRCLE('',#62181,10.);
#1174=CIRCLE('',#62182,10.);
#1175=CIRCLE('',#62183,10.);
#1176=CIRCLE('',#62184,10.);
#1177=CIRCLE('',#62185,10.);
#1178=CIRCLE('',#62186,10.);
#1179=CIRCLE('',#62187,10.);
#1180=CIRCLE('',#62188,10.);
#1181=CIRCLE('',#62190,10.);
#1182=CIRCLE('',#62192,10.);
#1183=CIRCLE('',#62196,10.);
#1184=CIRCLE('',#62198,9.2);
#1185=CIRCLE('',#62199,10.);
#1186=CIRCLE('',#62200,10.);
#1187=CIRCLE('',#62201,10.);
#1188=CIRCLE('',#62202,10.);
#1189=CIRCLE('',#62203,10.);
#1190=CIRCLE('',#62204,10.);
#1191=CIRCLE('',#62205,10.);
#1192=CIRCLE('',#62206,10.);
#1193=CIRCLE('',#62207,10.);
#1194=CIRCLE('',#62208,10.);
#1195=CIRCLE('',#62209,10.);
#1196=CIRCLE('',#62210,10.);
#1197=CIRCLE('',#62211,10.);
#1198=CIRCLE('',#62212,10.);
#1199=CIRCLE('',#62213,10.);
#1200=CIRCLE('',#62214,10.);
#1201=CIRCLE('',#62215,10.);
#1202=CIRCLE('',#62216,10.);
#1203=CIRCLE('',#62217,10.);
#1204=CIRCLE('',#62218,10.);
#1205=CIRCLE('',#62219,10.);
#1206=CIRCLE('',#62220,10.);
#1207=CIRCLE('',#62221,10.);
#1208=CIRCLE('',#62222,10.);
#1209=CIRCLE('',#62223,10.);
#1210=CIRCLE('',#62224,10.);
#1211=CIRCLE('',#62225,10.);
#1212=CIRCLE('',#62226,10.);
#1213=CIRCLE('',#62227,10.);
#1214=CIRCLE('',#62228,10.);
#1215=CIRCLE('',#62229,10.);
#1216=CIRCLE('',#62230,10.);
#1217=CIRCLE('',#62231,10.);
#1218=CIRCLE('',#62232,10.);
#1219=CIRCLE('',#62233,10.);
#1220=CIRCLE('',#62234,10.);
#1221=CIRCLE('',#62235,10.);
#1222=CIRCLE('',#62349,2.51000000000001);
#1223=CIRCLE('',#62350,2.81000000000001);
#1224=CIRCLE('',#62352,3.70000000000001);
#1225=CIRCLE('',#62354,4.);
#1226=CIRCLE('',#62356,4.);
#1227=CIRCLE('',#62358,4.40000000000001);
#1228=CIRCLE('',#62360,6.);
#1229=CIRCLE('',#62362,6.);
#1230=CIRCLE('',#62364,6.40000000000001);
#1231=CIRCLE('',#62368,7.4);
#1232=CIRCLE('',#62370,6.99999999999999);
#1233=CIRCLE('',#62373,2.51000000000001);
#1832=FACE_BOUND('',#9767,.T.);
#1833=FACE_BOUND('',#9772,.T.);
#1834=FACE_BOUND('',#9774,.T.);
#1835=FACE_BOUND('',#9777,.T.);
#1836=FACE_BOUND('',#9780,.T.);
#1837=FACE_BOUND('',#9785,.T.);
#3096=PLANE('',#62139);
#3097=PLANE('',#62144);
#3098=PLANE('',#62145);
#3099=PLANE('',#62146);
#3100=PLANE('',#62193);
#3101=PLANE('',#62194);
#3102=PLANE('',#62236);
#3103=PLANE('',#62237);
#3104=PLANE('',#62238);
#3105=PLANE('',#62239);
#3106=PLANE('',#62242);
#3107=PLANE('',#62243);
#3108=PLANE('',#62245);
#3109=PLANE('',#62246);
#3110=PLANE('',#62247);
#3111=PLANE('',#62248);
#3112=PLANE('',#62251);
#3113=PLANE('',#62252);
#3114=PLANE('',#62254);
#3115=PLANE('',#62255);
#3116=PLANE('',#62256);
#3117=PLANE('',#62257);
#3118=PLANE('',#62260);
#3119=PLANE('',#62261);
#3120=PLANE('',#62263);
#3121=PLANE('',#62264);
#3122=PLANE('',#62265);
#3123=PLANE('',#62266);
#3124=PLANE('',#62269);
#3125=PLANE('',#62270);
#3126=PLANE('',#62272);
#3127=PLANE('',#62273);
#3128=PLANE('',#62274);
#3129=PLANE('',#62275);
#3130=PLANE('',#62278);
#3131=PLANE('',#62279);
#3132=PLANE('',#62281);
#3133=PLANE('',#62282);
#3134=PLANE('',#62283);
#3135=PLANE('',#62284);
#3136=PLANE('',#62287);
#3137=PLANE('',#62288);
#3138=PLANE('',#62290);
#3139=PLANE('',#62291);
#3140=PLANE('',#62292);
#3141=PLANE('',#62293);
#3142=PLANE('',#62296);
#3143=PLANE('',#62297);
#3144=PLANE('',#62299);
#3145=PLANE('',#62300);
#3146=PLANE('',#62301);
#3147=PLANE('',#62302);
#3148=PLANE('',#62305);
#3149=PLANE('',#62306);
#3150=PLANE('',#62308);
#3151=PLANE('',#62309);
#3152=PLANE('',#62310);
#3153=PLANE('',#62311);
#3154=PLANE('',#62314);
#3155=PLANE('',#62315);
#3156=PLANE('',#62317);
#3157=PLANE('',#62318);
#3158=PLANE('',#62319);
#3159=PLANE('',#62320);
#3160=PLANE('',#62323);
#3161=PLANE('',#62324);
#3162=PLANE('',#62326);
#3163=PLANE('',#62327);
#3164=PLANE('',#62328);
#3165=PLANE('',#62329);
#3166=PLANE('',#62332);
#3167=PLANE('',#62333);
#3168=PLANE('',#62335);
#3169=PLANE('',#62336);
#3170=PLANE('',#62337);
#3171=PLANE('',#62338);
#3172=PLANE('',#62341);
#3173=PLANE('',#62342);
#3174=PLANE('',#62344);
#3175=PLANE('',#62345);
#3176=PLANE('',#62346);
#3177=PLANE('',#62347);
#3178=PLANE('',#62351);
#3179=PLANE('',#62359);
#3180=PLANE('',#62365);
#3181=PLANE('',#62367);
#3182=PLANE('',#62371);
#6084=FACE_OUTER_BOUND('',#9641,.T.);
#6085=FACE_OUTER_BOUND('',#9642,.T.);
#6086=FACE_OUTER_BOUND('',#9643,.T.);
#6087=FACE_OUTER_BOUND('',#9644,.T.);
#6088=FACE_OUTER_BOUND('',#9645,.T.);
#6089=FACE_OUTER_BOUND('',#9646,.T.);
#6090=FACE_OUTER_BOUND('',#9647,.T.);
#6091=FACE_OUTER_BOUND('',#9648,.T.);
#6092=FACE_OUTER_BOUND('',#9649,.T.);
#6093=FACE_OUTER_BOUND('',#9650,.T.);
#6094=FACE_OUTER_BOUND('',#9651,.T.);
#6095=FACE_OUTER_BOUND('',#9652,.T.);
#6096=FACE_OUTER_BOUND('',#9653,.T.);
#6097=FACE_OUTER_BOUND('',#9654,.T.);
#6098=FACE_OUTER_BOUND('',#9655,.T.);
#6099=FACE_OUTER_BOUND('',#9656,.T.);
#6100=FACE_OUTER_BOUND('',#9657,.T.);
#6101=FACE_OUTER_BOUND('',#9658,.T.);
#6102=FACE_OUTER_BOUND('',#9659,.T.);
#6103=FACE_OUTER_BOUND('',#9660,.T.);
#6104=FACE_OUTER_BOUND('',#9661,.T.);
#6105=FACE_OUTER_BOUND('',#9662,.T.);
#6106=FACE_OUTER_BOUND('',#9663,.T.);
#6107=FACE_OUTER_BOUND('',#9664,.T.);
#6108=FACE_OUTER_BOUND('',#9665,.T.);
#6109=FACE_OUTER_BOUND('',#9666,.T.);
#6110=FACE_OUTER_BOUND('',#9667,.T.);
#6111=FACE_OUTER_BOUND('',#9668,.T.);
#6112=FACE_OUTER_BOUND('',#9669,.T.);
#6113=FACE_OUTER_BOUND('',#9670,.T.);
#6114=FACE_OUTER_BOUND('',#9671,.T.);
#6115=FACE_OUTER_BOUND('',#9672,.T.);
#6116=FACE_OUTER_BOUND('',#9673,.T.);
#6117=FACE_OUTER_BOUND('',#9674,.T.);
#6118=FACE_OUTER_BOUND('',#9675,.T.);
#6119=FACE_OUTER_BOUND('',#9676,.T.);
#6120=FACE_OUTER_BOUND('',#9677,.T.);
#6121=FACE_OUTER_BOUND('',#9678,.T.);
#6122=FACE_OUTER_BOUND('',#9679,.T.);
#6123=FACE_OUTER_BOUND('',#9680,.T.);
#6124=FACE_OUTER_BOUND('',#9681,.T.);
#6125=FACE_OUTER_BOUND('',#9682,.T.);
#6126=FACE_OUTER_BOUND('',#9683,.T.);
#6127=FACE_OUTER_BOUND('',#9684,.T.);
#6128=FACE_OUTER_BOUND('',#9685,.T.);
#6129=FACE_OUTER_BOUND('',#9686,.T.);
#6130=FACE_OUTER_BOUND('',#9687,.T.);
#6131=FACE_OUTER_BOUND('',#9688,.T.);
#6132=FACE_OUTER_BOUND('',#9689,.T.);
#6133=FACE_OUTER_BOUND('',#9690,.T.);
#6134=FACE_OUTER_BOUND('',#9691,.T.);
#6135=FACE_OUTER_BOUND('',#9692,.T.);
#6136=FACE_OUTER_BOUND('',#9693,.T.);
#6137=FACE_OUTER_BOUND('',#9694,.T.);
#6138=FACE_OUTER_BOUND('',#9695,.T.);
#6139=FACE_OUTER_BOUND('',#9696,.T.);
#6140=FACE_OUTER_BOUND('',#9697,.T.);
#6141=FACE_OUTER_BOUND('',#9698,.T.);
#6142=FACE_OUTER_BOUND('',#9699,.T.);
#6143=FACE_OUTER_BOUND('',#9700,.T.);
#6144=FACE_OUTER_BOUND('',#9701,.T.);
#6145=FACE_OUTER_BOUND('',#9702,.T.);
#6146=FACE_OUTER_BOUND('',#9703,.T.);
#6147=FACE_OUTER_BOUND('',#9704,.T.);
#6148=FACE_OUTER_BOUND('',#9705,.T.);
#6149=FACE_OUTER_BOUND('',#9706,.T.);
#6150=FACE_OUTER_BOUND('',#9707,.T.);
#6151=FACE_OUTER_BOUND('',#9708,.T.);
#6152=FACE_OUTER_BOUND('',#9709,.T.);
#6153=FACE_OUTER_BOUND('',#9710,.T.);
#6154=FACE_OUTER_BOUND('',#9711,.T.);
#6155=FACE_OUTER_BOUND('',#9712,.T.);
#6156=FACE_OUTER_BOUND('',#9713,.T.);
#6157=FACE_OUTER_BOUND('',#9714,.T.);
#6158=FACE_OUTER_BOUND('',#9715,.T.);
#6159=FACE_OUTER_BOUND('',#9716,.T.);
#6160=FACE_OUTER_BOUND('',#9717,.T.);
#6161=FACE_OUTER_BOUND('',#9718,.T.);
#6162=FACE_OUTER_BOUND('',#9719,.T.);
#6163=FACE_OUTER_BOUND('',#9720,.T.);
#6164=FACE_OUTER_BOUND('',#9721,.T.);
#6165=FACE_OUTER_BOUND('',#9722,.T.);
#6166=FACE_OUTER_BOUND('',#9723,.T.);
#6167=FACE_OUTER_BOUND('',#9724,.T.);
#6168=FACE_OUTER_BOUND('',#9725,.T.);
#6169=FACE_OUTER_BOUND('',#9726,.T.);
#6170=FACE_OUTER_BOUND('',#9727,.T.);
#6171=FACE_OUTER_BOUND('',#9728,.T.);
#6172=FACE_OUTER_BOUND('',#9729,.T.);
#6173=FACE_OUTER_BOUND('',#9730,.T.);
#6174=FACE_OUTER_BOUND('',#9731,.T.);
#6175=FACE_OUTER_BOUND('',#9732,.T.);
#6176=FACE_OUTER_BOUND('',#9733,.T.);
#6177=FACE_OUTER_BOUND('',#9734,.T.);
#6178=FACE_OUTER_BOUND('',#9735,.T.);
#6179=FACE_OUTER_BOUND('',#9736,.T.);
#6180=FACE_OUTER_BOUND('',#9737,.T.);
#6181=FACE_OUTER_BOUND('',#9738,.T.);
#6182=FACE_OUTER_BOUND('',#9739,.T.);
#6183=FACE_OUTER_BOUND('',#9740,.T.);
#6184=FACE_OUTER_BOUND('',#9741,.T.);
#6185=FACE_OUTER_BOUND('',#9742,.T.);
#6186=FACE_OUTER_BOUND('',#9743,.T.);
#6187=FACE_OUTER_BOUND('',#9744,.T.);
#6188=FACE_OUTER_BOUND('',#9745,.T.);
#6189=FACE_OUTER_BOUND('',#9746,.T.);
#6190=FACE_OUTER_BOUND('',#9747,.T.);
#6191=FACE_OUTER_BOUND('',#9748,.T.);
#6192=FACE_OUTER_BOUND('',#9749,.T.);
#6193=FACE_OUTER_BOUND('',#9750,.T.);
#6194=FACE_OUTER_BOUND('',#9751,.T.);
#6195=FACE_OUTER_BOUND('',#9752,.T.);
#6196=FACE_OUTER_BOUND('',#9753,.T.);
#6197=FACE_OUTER_BOUND('',#9754,.T.);
#6198=FACE_OUTER_BOUND('',#9755,.T.);
#6199=FACE_OUTER_BOUND('',#9756,.T.);
#6200=FACE_OUTER_BOUND('',#9757,.T.);
#6201=FACE_OUTER_BOUND('',#9758,.T.);
#6202=FACE_OUTER_BOUND('',#9759,.T.);
#6203=FACE_OUTER_BOUND('',#9760,.T.);
#6204=FACE_OUTER_BOUND('',#9761,.T.);
#6205=FACE_OUTER_BOUND('',#9762,.T.);
#6206=FACE_OUTER_BOUND('',#9763,.T.);
#6207=FACE_OUTER_BOUND('',#9764,.T.);
#6208=FACE_OUTER_BOUND('',#9765,.T.);
#6209=FACE_OUTER_BOUND('',#9766,.T.);
#6210=FACE_OUTER_BOUND('',#9768,.T.);
#6211=FACE_OUTER_BOUND('',#9769,.T.);
#6212=FACE_OUTER_BOUND('',#9770,.T.);
#6213=FACE_OUTER_BOUND('',#9771,.T.);
#6214=FACE_OUTER_BOUND('',#9773,.T.);
#6215=FACE_OUTER_BOUND('',#9775,.T.);
#6216=FACE_OUTER_BOUND('',#9776,.T.);
#6217=FACE_OUTER_BOUND('',#9778,.T.);
#6218=FACE_OUTER_BOUND('',#9779,.T.);
#6219=FACE_OUTER_BOUND('',#9781,.T.);
#6220=FACE_OUTER_BOUND('',#9782,.T.);
#6221=FACE_OUTER_BOUND('',#9783,.T.);
#6222=FACE_OUTER_BOUND('',#9784,.T.);
#9641=EDGE_LOOP('',(#49607,#49608,#49609));
#9642=EDGE_LOOP('',(#49610,#49611,#49612,#49613,#49614,#49615,#49616,#49617,
#49618,#49619));
#9643=EDGE_LOOP('',(#49620,#49621));
#9644=EDGE_LOOP('',(#49622,#49623,#49624,#49625));
#9645=EDGE_LOOP('',(#49626,#49627,#49628,#49629));
#9646=EDGE_LOOP('',(#49630,#49631,#49632,#49633,#49634,#49635,#49636,#49637,
#49638,#49639,#49640,#49641,#49642,#49643,#49644,#49645,#49646,#49647,#49648,
#49649,#49650,#49651,#49652,#49653,#49654,#49655,#49656,#49657,#49658,#49659,
#49660,#49661,#49662,#49663,#49664,#49665,#49666,#49667,#49668,#49669,#49670,
#49671,#49672,#49673,#49674,#49675,#49676,#49677,#49678,#49679,#49680,#49681,
#49682,#49683,#49684,#49685,#49686,#49687,#49688,#49689,#49690,#49691,#49692,
#49693,#49694,#49695,#49696,#49697,#49698,#49699,#49700,#49701,#49702,#49703,
#49704,#49705,#49706,#49707,#49708,#49709,#49710,#49711,#49712,#49713,#49714,
#49715,#49716,#49717,#49718,#49719,#49720,#49721,#49722,#49723,#49724,#49725,
#49726,#49727,#49728,#49729,#49730,#49731,#49732,#49733,#49734,#49735,#49736,
#49737,#49738,#49739,#49740,#49741,#49742,#49743,#49744,#49745,#49746,#49747,
#49748,#49749,#49750,#49751,#49752));
#9647=EDGE_LOOP('',(#49753,#49754,#49755,#49756));
#9648=EDGE_LOOP('',(#49757,#49758,#49759,#49760));
#9649=EDGE_LOOP('',(#49761,#49762,#49763,#49764));
#9650=EDGE_LOOP('',(#49765,#49766,#49767,#49768));
#9651=EDGE_LOOP('',(#49769,#49770,#49771,#49772));
#9652=EDGE_LOOP('',(#49773,#49774,#49775,#49776,#49777,#49778,#49779,#49780,
#49781,#49782,#49783,#49784,#49785,#49786,#49787,#49788,#49789,#49790,#49791,
#49792,#49793,#49794,#49795,#49796,#49797,#49798,#49799,#49800,#49801,#49802,
#49803,#49804,#49805,#49806,#49807,#49808,#49809,#49810,#49811,#49812,#49813,
#49814,#49815,#49816,#49817,#49818,#49819,#49820,#49821,#49822,#49823,#49824,
#49825,#49826,#49827,#49828,#49829,#49830,#49831,#49832,#49833,#49834,#49835,
#49836,#49837,#49838,#49839,#49840,#49841,#49842,#49843,#49844,#49845,#49846,
#49847,#49848,#49849,#49850,#49851,#49852,#49853,#49854,#49855,#49856,#49857,
#49858,#49859,#49860,#49861,#49862,#49863,#49864,#49865,#49866,#49867,#49868,
#49869,#49870,#49871,#49872,#49873,#49874,#49875,#49876,#49877,#49878,#49879,
#49880,#49881,#49882,#49883,#49884,#49885,#49886,#49887,#49888,#49889,#49890,
#49891,#49892,#49893,#49894,#49895));
#9653=EDGE_LOOP('',(#49896,#49897,#49898,#49899));
#9654=EDGE_LOOP('',(#49900,#49901,#49902,#49903));
#9655=EDGE_LOOP('',(#49904,#49905,#49906,#49907));
#9656=EDGE_LOOP('',(#49908,#49909,#49910,#49911));
#9657=EDGE_LOOP('',(#49912,#49913,#49914,#49915));
#9658=EDGE_LOOP('',(#49916,#49917,#49918,#49919));
#9659=EDGE_LOOP('',(#49920,#49921,#49922,#49923));
#9660=EDGE_LOOP('',(#49924,#49925,#49926,#49927));
#9661=EDGE_LOOP('',(#49928,#49929,#49930,#49931));
#9662=EDGE_LOOP('',(#49932,#49933,#49934,#49935));
#9663=EDGE_LOOP('',(#49936,#49937,#49938,#49939));
#9664=EDGE_LOOP('',(#49940,#49941,#49942,#49943));
#9665=EDGE_LOOP('',(#49944,#49945,#49946,#49947));
#9666=EDGE_LOOP('',(#49948,#49949,#49950,#49951));
#9667=EDGE_LOOP('',(#49952,#49953,#49954,#49955));
#9668=EDGE_LOOP('',(#49956,#49957,#49958,#49959));
#9669=EDGE_LOOP('',(#49960,#49961,#49962,#49963));
#9670=EDGE_LOOP('',(#49964,#49965,#49966,#49967));
#9671=EDGE_LOOP('',(#49968,#49969,#49970,#49971));
#9672=EDGE_LOOP('',(#49972,#49973,#49974,#49975));
#9673=EDGE_LOOP('',(#49976,#49977,#49978,#49979));
#9674=EDGE_LOOP('',(#49980,#49981,#49982,#49983));
#9675=EDGE_LOOP('',(#49984,#49985,#49986,#49987));
#9676=EDGE_LOOP('',(#49988,#49989,#49990,#49991));
#9677=EDGE_LOOP('',(#49992,#49993,#49994,#49995));
#9678=EDGE_LOOP('',(#49996,#49997,#49998,#49999));
#9679=EDGE_LOOP('',(#50000,#50001,#50002,#50003));
#9680=EDGE_LOOP('',(#50004,#50005,#50006,#50007));
#9681=EDGE_LOOP('',(#50008,#50009,#50010,#50011));
#9682=EDGE_LOOP('',(#50012,#50013,#50014,#50015));
#9683=EDGE_LOOP('',(#50016,#50017,#50018,#50019));
#9684=EDGE_LOOP('',(#50020,#50021,#50022,#50023));
#9685=EDGE_LOOP('',(#50024,#50025,#50026,#50027));
#9686=EDGE_LOOP('',(#50028,#50029,#50030,#50031));
#9687=EDGE_LOOP('',(#50032,#50033,#50034,#50035));
#9688=EDGE_LOOP('',(#50036,#50037,#50038,#50039));
#9689=EDGE_LOOP('',(#50040,#50041,#50042,#50043));
#9690=EDGE_LOOP('',(#50044,#50045,#50046,#50047));
#9691=EDGE_LOOP('',(#50048,#50049,#50050,#50051));
#9692=EDGE_LOOP('',(#50052,#50053,#50054,#50055));
#9693=EDGE_LOOP('',(#50056,#50057,#50058,#50059));
#9694=EDGE_LOOP('',(#50060,#50061,#50062,#50063));
#9695=EDGE_LOOP('',(#50064,#50065,#50066,#50067));
#9696=EDGE_LOOP('',(#50068,#50069,#50070,#50071));
#9697=EDGE_LOOP('',(#50072,#50073,#50074,#50075));
#9698=EDGE_LOOP('',(#50076,#50077,#50078,#50079));
#9699=EDGE_LOOP('',(#50080,#50081,#50082,#50083));
#9700=EDGE_LOOP('',(#50084,#50085,#50086,#50087));
#9701=EDGE_LOOP('',(#50088,#50089,#50090,#50091));
#9702=EDGE_LOOP('',(#50092,#50093,#50094,#50095));
#9703=EDGE_LOOP('',(#50096,#50097,#50098,#50099));
#9704=EDGE_LOOP('',(#50100,#50101,#50102,#50103));
#9705=EDGE_LOOP('',(#50104,#50105,#50106,#50107));
#9706=EDGE_LOOP('',(#50108,#50109,#50110,#50111));
#9707=EDGE_LOOP('',(#50112,#50113,#50114,#50115));
#9708=EDGE_LOOP('',(#50116,#50117,#50118,#50119));
#9709=EDGE_LOOP('',(#50120,#50121,#50122,#50123));
#9710=EDGE_LOOP('',(#50124,#50125,#50126,#50127));
#9711=EDGE_LOOP('',(#50128,#50129,#50130,#50131));
#9712=EDGE_LOOP('',(#50132,#50133,#50134,#50135));
#9713=EDGE_LOOP('',(#50136,#50137,#50138,#50139));
#9714=EDGE_LOOP('',(#50140,#50141,#50142,#50143));
#9715=EDGE_LOOP('',(#50144,#50145,#50146,#50147));
#9716=EDGE_LOOP('',(#50148,#50149,#50150,#50151));
#9717=EDGE_LOOP('',(#50152,#50153,#50154,#50155));
#9718=EDGE_LOOP('',(#50156,#50157,#50158,#50159));
#9719=EDGE_LOOP('',(#50160,#50161,#50162,#50163));
#9720=EDGE_LOOP('',(#50164,#50165,#50166,#50167));
#9721=EDGE_LOOP('',(#50168,#50169,#50170,#50171));
#9722=EDGE_LOOP('',(#50172,#50173,#50174,#50175));
#9723=EDGE_LOOP('',(#50176,#50177,#50178,#50179));
#9724=EDGE_LOOP('',(#50180,#50181,#50182,#50183));
#9725=EDGE_LOOP('',(#50184,#50185,#50186,#50187));
#9726=EDGE_LOOP('',(#50188,#50189,#50190,#50191));
#9727=EDGE_LOOP('',(#50192,#50193,#50194,#50195));
#9728=EDGE_LOOP('',(#50196,#50197,#50198,#50199));
#9729=EDGE_LOOP('',(#50200,#50201,#50202,#50203));
#9730=EDGE_LOOP('',(#50204,#50205,#50206,#50207));
#9731=EDGE_LOOP('',(#50208,#50209,#50210,#50211));
#9732=EDGE_LOOP('',(#50212,#50213,#50214,#50215));
#9733=EDGE_LOOP('',(#50216,#50217,#50218,#50219));
#9734=EDGE_LOOP('',(#50220,#50221,#50222,#50223));
#9735=EDGE_LOOP('',(#50224,#50225,#50226,#50227));
#9736=EDGE_LOOP('',(#50228,#50229,#50230,#50231));
#9737=EDGE_LOOP('',(#50232,#50233,#50234,#50235));
#9738=EDGE_LOOP('',(#50236,#50237,#50238,#50239));
#9739=EDGE_LOOP('',(#50240,#50241,#50242,#50243));
#9740=EDGE_LOOP('',(#50244,#50245,#50246,#50247));
#9741=EDGE_LOOP('',(#50248,#50249,#50250,#50251));
#9742=EDGE_LOOP('',(#50252,#50253,#50254,#50255));
#9743=EDGE_LOOP('',(#50256,#50257,#50258,#50259));
#9744=EDGE_LOOP('',(#50260,#50261,#50262,#50263));
#9745=EDGE_LOOP('',(#50264,#50265,#50266,#50267));
#9746=EDGE_LOOP('',(#50268,#50269,#50270,#50271));
#9747=EDGE_LOOP('',(#50272,#50273,#50274,#50275));
#9748=EDGE_LOOP('',(#50276,#50277,#50278,#50279));
#9749=EDGE_LOOP('',(#50280,#50281,#50282,#50283));
#9750=EDGE_LOOP('',(#50284,#50285,#50286,#50287));
#9751=EDGE_LOOP('',(#50288,#50289,#50290,#50291));
#9752=EDGE_LOOP('',(#50292,#50293,#50294,#50295));
#9753=EDGE_LOOP('',(#50296,#50297,#50298,#50299));
#9754=EDGE_LOOP('',(#50300,#50301,#50302,#50303));
#9755=EDGE_LOOP('',(#50304,#50305,#50306,#50307));
#9756=EDGE_LOOP('',(#50308,#50309,#50310,#50311));
#9757=EDGE_LOOP('',(#50312,#50313,#50314,#50315));
#9758=EDGE_LOOP('',(#50316,#50317,#50318,#50319));
#9759=EDGE_LOOP('',(#50320,#50321,#50322,#50323));
#9760=EDGE_LOOP('',(#50324,#50325,#50326,#50327));
#9761=EDGE_LOOP('',(#50328,#50329,#50330,#50331));
#9762=EDGE_LOOP('',(#50332,#50333,#50334,#50335));
#9763=EDGE_LOOP('',(#50336,#50337,#50338,#50339));
#9764=EDGE_LOOP('',(#50340,#50341,#50342,#50343));
#9765=EDGE_LOOP('',(#50344,#50345,#50346,#50347));
#9766=EDGE_LOOP('',(#50348));
#9767=EDGE_LOOP('',(#50349));
#9768=EDGE_LOOP('',(#50350,#50351,#50352,#50353));
#9769=EDGE_LOOP('',(#50354,#50355,#50356,#50357));
#9770=EDGE_LOOP('',(#50358,#50359,#50360,#50361));
#9771=EDGE_LOOP('',(#50362));
#9772=EDGE_LOOP('',(#50363));
#9773=EDGE_LOOP('',(#50364,#50365,#50366,#50367));
#9774=EDGE_LOOP('',(#50368,#50369,#50370));
#9775=EDGE_LOOP('',(#50371,#50372,#50373,#50374));
#9776=EDGE_LOOP('',(#50375));
#9777=EDGE_LOOP('',(#50376));
#9778=EDGE_LOOP('',(#50377,#50378,#50379,#50380));
#9779=EDGE_LOOP('',(#50381));
#9780=EDGE_LOOP('',(#50382));
#9781=EDGE_LOOP('',(#50383,#50384,#50385,#50386));
#9782=EDGE_LOOP('',(#50387));
#9783=EDGE_LOOP('',(#50388,#50389,#50390));
#9784=EDGE_LOOP('',(#50391,#50392,#50393,#50394));
#9785=EDGE_LOOP('',(#50395,#50396,#50397,#50398));
#14496=LINE('',#97722,#20530);
#14497=LINE('',#97769,#20531);
#14498=LINE('',#97810,#20532);
#14499=LINE('',#97818,#20533);
#14500=LINE('',#97823,#20534);
#14501=LINE('',#97830,#20535);
#14502=LINE('',#98022,#20536);
#14503=LINE('',#98232,#20537);
#14504=LINE('',#98235,#20538);
#14505=LINE('',#98239,#20539);
#14506=LINE('',#98244,#20540);
#14507=LINE('',#98252,#20541);
#14508=LINE('',#98257,#20542);
#14509=LINE('',#98635,#20543);
#14510=LINE('',#98637,#20544);
#14511=LINE('',#98639,#20545);
#14512=LINE('',#98640,#20546);
#14513=LINE('',#98642,#20547);
#14514=LINE('',#98644,#20548);
#14515=LINE('',#98647,#20549);
#14516=LINE('',#98648,#20550);
#14517=LINE('',#98651,#20551);
#14518=LINE('',#98653,#20552);
#14519=LINE('',#98655,#20553);
#14520=LINE('',#98657,#20554);
#14521=LINE('',#98658,#20555);
#14522=LINE('',#98660,#20556);
#14523=LINE('',#98662,#20557);
#14524=LINE('',#98665,#20558);
#14525=LINE('',#98666,#20559);
#14526=LINE('',#98669,#20560);
#14527=LINE('',#98671,#20561);
#14528=LINE('',#98673,#20562);
#14529=LINE('',#98675,#20563);
#14530=LINE('',#98676,#20564);
#14531=LINE('',#98678,#20565);
#14532=LINE('',#98680,#20566);
#14533=LINE('',#98683,#20567);
#14534=LINE('',#98684,#20568);
#14535=LINE('',#98687,#20569);
#14536=LINE('',#98689,#20570);
#14537=LINE('',#98691,#20571);
#14538=LINE('',#98693,#20572);
#14539=LINE('',#98694,#20573);
#14540=LINE('',#98696,#20574);
#14541=LINE('',#98698,#20575);
#14542=LINE('',#98701,#20576);
#14543=LINE('',#98702,#20577);
#14544=LINE('',#98705,#20578);
#14545=LINE('',#98707,#20579);
#14546=LINE('',#98709,#20580);
#14547=LINE('',#98711,#20581);
#14548=LINE('',#98712,#20582);
#14549=LINE('',#98714,#20583);
#14550=LINE('',#98716,#20584);
#14551=LINE('',#98719,#20585);
#14552=LINE('',#98720,#20586);
#14553=LINE('',#98723,#20587);
#14554=LINE('',#98725,#20588);
#14555=LINE('',#98727,#20589);
#14556=LINE('',#98729,#20590);
#14557=LINE('',#98730,#20591);
#14558=LINE('',#98732,#20592);
#14559=LINE('',#98734,#20593);
#14560=LINE('',#98737,#20594);
#14561=LINE('',#98738,#20595);
#14562=LINE('',#98741,#20596);
#14563=LINE('',#98743,#20597);
#14564=LINE('',#98745,#20598);
#14565=LINE('',#98747,#20599);
#14566=LINE('',#98748,#20600);
#14567=LINE('',#98750,#20601);
#14568=LINE('',#98752,#20602);
#14569=LINE('',#98755,#20603);
#14570=LINE('',#98756,#20604);
#14571=LINE('',#98759,#20605);
#14572=LINE('',#98761,#20606);
#14573=LINE('',#98763,#20607);
#14574=LINE('',#98765,#20608);
#14575=LINE('',#98766,#20609);
#14576=LINE('',#98768,#20610);
#14577=LINE('',#98770,#20611);
#14578=LINE('',#98773,#20612);
#14579=LINE('',#98774,#20613);
#14580=LINE('',#98777,#20614);
#14581=LINE('',#98779,#20615);
#14582=LINE('',#98781,#20616);
#14583=LINE('',#98783,#20617);
#14584=LINE('',#98784,#20618);
#14585=LINE('',#98786,#20619);
#14586=LINE('',#98788,#20620);
#14587=LINE('',#98791,#20621);
#14588=LINE('',#98792,#20622);
#14589=LINE('',#98795,#20623);
#14590=LINE('',#98797,#20624);
#14591=LINE('',#98799,#20625);
#14592=LINE('',#98801,#20626);
#14593=LINE('',#98802,#20627);
#14594=LINE('',#98804,#20628);
#14595=LINE('',#98806,#20629);
#14596=LINE('',#98809,#20630);
#14597=LINE('',#98810,#20631);
#14598=LINE('',#98813,#20632);
#14599=LINE('',#98815,#20633);
#14600=LINE('',#98817,#20634);
#14601=LINE('',#98819,#20635);
#14602=LINE('',#98820,#20636);
#14603=LINE('',#98822,#20637);
#14604=LINE('',#98824,#20638);
#14605=LINE('',#98827,#20639);
#14606=LINE('',#98828,#20640);
#14607=LINE('',#98831,#20641);
#14608=LINE('',#98833,#20642);
#14609=LINE('',#98835,#20643);
#14610=LINE('',#98837,#20644);
#14611=LINE('',#98838,#20645);
#14612=LINE('',#98840,#20646);
#14613=LINE('',#98842,#20647);
#14614=LINE('',#98845,#20648);
#14615=LINE('',#98846,#20649);
#14616=LINE('',#98849,#20650);
#14617=LINE('',#98851,#20651);
#14618=LINE('',#98853,#20652);
#14619=LINE('',#98855,#20653);
#14620=LINE('',#98856,#20654);
#14621=LINE('',#98862,#20655);
#14622=LINE('',#98870,#20656);
#14623=LINE('',#98874,#20657);
#14624=LINE('',#98878,#20658);
#14625=LINE('',#98885,#20659);
#14626=LINE('',#98889,#20660);
#14627=LINE('',#98897,#20661);
#14628=LINE('',#98903,#20662);
#14629=LINE('',#98906,#20663);
#20530=VECTOR('',#70458,10.);
#20531=VECTOR('',#70465,1.54999999999999);
#20532=VECTOR('',#70470,10.);
#20533=VECTOR('',#70473,10.);
#20534=VECTOR('',#70474,10.);
#20535=VECTOR('',#70477,10.);
#20536=VECTOR('',#70518,9.60000000000001);
#20537=VECTOR('',#70567,10.);
#20538=VECTOR('',#70570,10.);
#20539=VECTOR('',#70575,10.);
#20540=VECTOR('',#70576,10.);
#20541=VECTOR('',#70583,10.);
#20542=VECTOR('',#70588,9.60000000000001);
#20543=VECTOR('',#70665,10.);
#20544=VECTOR('',#70668,10.);
#20545=VECTOR('',#70671,10.);
#20546=VECTOR('',#70672,10.);
#20547=VECTOR('',#70675,10.);
#20548=VECTOR('',#70678,10.);
#20549=VECTOR('',#70683,10.);
#20550=VECTOR('',#70684,10.);
#20551=VECTOR('',#70689,10.);
#20552=VECTOR('',#70692,10.);
#20553=VECTOR('',#70695,10.);
#20554=VECTOR('',#70698,10.);
#20555=VECTOR('',#70699,10.);
#20556=VECTOR('',#70702,10.);
#20557=VECTOR('',#70705,10.);
#20558=VECTOR('',#70710,10.);
#20559=VECTOR('',#70711,10.);
#20560=VECTOR('',#70716,10.);
#20561=VECTOR('',#70719,10.);
#20562=VECTOR('',#70722,10.);
#20563=VECTOR('',#70725,10.);
#20564=VECTOR('',#70726,10.);
#20565=VECTOR('',#70729,10.);
#20566=VECTOR('',#70732,10.);
#20567=VECTOR('',#70737,10.);
#20568=VECTOR('',#70738,10.);
#20569=VECTOR('',#70743,10.);
#20570=VECTOR('',#70746,10.);
#20571=VECTOR('',#70749,10.);
#20572=VECTOR('',#70752,10.);
#20573=VECTOR('',#70753,10.);
#20574=VECTOR('',#70756,10.);
#20575=VECTOR('',#70759,10.);
#20576=VECTOR('',#70764,10.);
#20577=VECTOR('',#70765,10.);
#20578=VECTOR('',#70770,10.);
#20579=VECTOR('',#70773,10.);
#20580=VECTOR('',#70776,10.);
#20581=VECTOR('',#70779,10.);
#20582=VECTOR('',#70780,10.);
#20583=VECTOR('',#70783,10.);
#20584=VECTOR('',#70786,10.);
#20585=VECTOR('',#70791,10.);
#20586=VECTOR('',#70792,10.);
#20587=VECTOR('',#70797,10.);
#20588=VECTOR('',#70800,10.);
#20589=VECTOR('',#70803,10.);
#20590=VECTOR('',#70806,10.);
#20591=VECTOR('',#70807,10.);
#20592=VECTOR('',#70810,10.);
#20593=VECTOR('',#70813,10.);
#20594=VECTOR('',#70818,10.);
#20595=VECTOR('',#70819,10.);
#20596=VECTOR('',#70824,10.);
#20597=VECTOR('',#70827,10.);
#20598=VECTOR('',#70830,10.);
#20599=VECTOR('',#70833,10.);
#20600=VECTOR('',#70834,10.);
#20601=VECTOR('',#70837,10.);
#20602=VECTOR('',#70840,10.);
#20603=VECTOR('',#70845,10.);
#20604=VECTOR('',#70846,10.);
#20605=VECTOR('',#70851,10.);
#20606=VECTOR('',#70854,10.);
#20607=VECTOR('',#70857,10.);
#20608=VECTOR('',#70860,10.);
#20609=VECTOR('',#70861,10.);
#20610=VECTOR('',#70864,10.);
#20611=VECTOR('',#70867,10.);
#20612=VECTOR('',#70872,10.);
#20613=VECTOR('',#70873,10.);
#20614=VECTOR('',#70878,10.);
#20615=VECTOR('',#70881,10.);
#20616=VECTOR('',#70884,10.);
#20617=VECTOR('',#70887,10.);
#20618=VECTOR('',#70888,10.);
#20619=VECTOR('',#70891,10.);
#20620=VECTOR('',#70894,10.);
#20621=VECTOR('',#70899,10.);
#20622=VECTOR('',#70900,10.);
#20623=VECTOR('',#70905,10.);
#20624=VECTOR('',#70908,10.);
#20625=VECTOR('',#70911,10.);
#20626=VECTOR('',#70914,10.);
#20627=VECTOR('',#70915,10.);
#20628=VECTOR('',#70918,10.);
#20629=VECTOR('',#70921,10.);
#20630=VECTOR('',#70926,10.);
#20631=VECTOR('',#70927,10.);
#20632=VECTOR('',#70932,10.);
#20633=VECTOR('',#70935,10.);
#20634=VECTOR('',#70938,10.);
#20635=VECTOR('',#70941,10.);
#20636=VECTOR('',#70942,10.);
#20637=VECTOR('',#70945,10.);
#20638=VECTOR('',#70948,10.);
#20639=VECTOR('',#70953,10.);
#20640=VECTOR('',#70954,10.);
#20641=VECTOR('',#70959,10.);
#20642=VECTOR('',#70962,10.);
#20643=VECTOR('',#70965,10.);
#20644=VECTOR('',#70968,10.);
#20645=VECTOR('',#70969,10.);
#20646=VECTOR('',#70972,10.);
#20647=VECTOR('',#70975,10.);
#20648=VECTOR('',#70980,10.);
#20649=VECTOR('',#70981,10.);
#20650=VECTOR('',#70986,10.);
#20651=VECTOR('',#70989,10.);
#20652=VECTOR('',#70992,10.);
#20653=VECTOR('',#70995,10.);
#20654=VECTOR('',#70996,10.);
#20655=VECTOR('',#71003,2.66000000000002);
#20656=VECTOR('',#71014,3.85000000000002);
#20657=VECTOR('',#71019,4.);
#20658=VECTOR('',#71024,4.20000000000002);
#20659=VECTOR('',#71033,6.);
#20660=VECTOR('',#71038,6.20000000000001);
#20661=VECTOR('',#71049,7.19999999999999);
#20662=VECTOR('',#71056,1.25500000000001);
#20663=VECTOR('',#71061,2.51000000000001);
#24345=B_SPLINE_CURVE_WITH_KNOTS('',3,(#97729,#97730,#97731,#97732,#97733,
#97734,#97735,#97736,#97737,#97738),.UNSPECIFIED.,.F.,.F.,(4,2,2,2,4),(0.234696888241094,
0.293366413777628,0.352035939314162,0.410714857898175,0.469393776482188),
 .UNSPECIFIED.);
#24346=B_SPLINE_CURVE_WITH_KNOTS('',3,(#97740,#97741,#97742,#97743,#97744,
#97745,#97746,#97747,#97748,#97749,#97750,#97751,#97752,#97753,#97754,#97755,
#97756,#97757,#97758),.UNSPECIFIED.,.F.,.F.,(4,2,2,2,3,2,2,2,4),(0.704090664723282,
0.762760190259816,0.82142971579635,0.880108634380363,0.938787552964375,
0.997466471548388,1.0561453901324,1.11481491566894,1.17348444120547),
 .UNSPECIFIED.);
#24347=B_SPLINE_CURVE_WITH_KNOTS('',3,(#97759,#97760,#97761,#97762,#97763,
#97764,#97765,#97766,#97767,#97768),.UNSPECIFIED.,.F.,.F.,(4,2,2,2,4),(0.469393776482188,
0.5280726950662,0.586751613650213,0.645421139186747,0.704090664723282),
 .UNSPECIFIED.);
#24348=B_SPLINE_CURVE_WITH_KNOTS('',3,(#97771,#97772,#97773,#97774,#97775,
#97776,#97777,#97778,#97779,#97780,#97781,#97782,#97783,#97784,#97785,#97786,
#97787,#97788),.UNSPECIFIED.,.F.,.F.,(4,2,2,2,2,2,2,2,4),(0.0317636912176915,
0.0605992517752672,0.121198503550534,0.181346844389925,0.241495185229315,
0.301643526068706,0.361791866908096,0.422391118683363,0.45122667924094),
 .UNSPECIFIED.);
#24349=B_SPLINE_CURVE_WITH_KNOTS('',3,(#97791,#97792,#97793,#97794,#97795,
#97796,#97797,#97798,#97799,#97800,#97801,#97802,#97803,#97804,#97805,#97806,
#97807,#97808),.UNSPECIFIED.,.F.,.F.,(4,2,2,2,2,2,2,2,4),(0.514754061676322,
0.543589622233898,0.604188874009165,0.664337214848555,0.724485555687945,
0.784633896527336,0.844782237366726,0.905381489141993,0.934217049699569),
 .UNSPECIFIED.);
#28118=VERTEX_POINT('',#97720);
#28119=VERTEX_POINT('',#97721);
#28120=VERTEX_POINT('',#97723);
#28121=VERTEX_POINT('',#97727);
#28122=VERTEX_POINT('',#97728);
#28123=VERTEX_POINT('',#97739);
#28124=VERTEX_POINT('',#97770);
#28125=VERTEX_POINT('',#97789);
#28126=VERTEX_POINT('',#97812);
#28127=VERTEX_POINT('',#97813);
#28128=VERTEX_POINT('',#97817);
#28129=VERTEX_POINT('',#97819);
#28130=VERTEX_POINT('',#97825);
#28131=VERTEX_POINT('',#97829);
#28132=VERTEX_POINT('',#97835);
#28133=VERTEX_POINT('',#97837);
#28134=VERTEX_POINT('',#97841);
#28135=VERTEX_POINT('',#97845);
#28136=VERTEX_POINT('',#97847);
#28137=VERTEX_POINT('',#97851);
#28138=VERTEX_POINT('',#97855);
#28139=VERTEX_POINT('',#97857);
#28140=VERTEX_POINT('',#97861);
#28141=VERTEX_POINT('',#97865);
#28142=VERTEX_POINT('',#97867);
#28143=VERTEX_POINT('',#97871);
#28144=VERTEX_POINT('',#97875);
#28145=VERTEX_POINT('',#97877);
#28146=VERTEX_POINT('',#97881);
#28147=VERTEX_POINT('',#97885);
#28148=VERTEX_POINT('',#97887);
#28149=VERTEX_POINT('',#97891);
#28150=VERTEX_POINT('',#97895);
#28151=VERTEX_POINT('',#97897);
#28152=VERTEX_POINT('',#97901);
#28153=VERTEX_POINT('',#97905);
#28154=VERTEX_POINT('',#97907);
#28155=VERTEX_POINT('',#97911);
#28156=VERTEX_POINT('',#97915);
#28157=VERTEX_POINT('',#97917);
#28158=VERTEX_POINT('',#97921);
#28159=VERTEX_POINT('',#97925);
#28160=VERTEX_POINT('',#97927);
#28161=VERTEX_POINT('',#97931);
#28162=VERTEX_POINT('',#97935);
#28163=VERTEX_POINT('',#97937);
#28164=VERTEX_POINT('',#97941);
#28165=VERTEX_POINT('',#97945);
#28166=VERTEX_POINT('',#97947);
#28167=VERTEX_POINT('',#97951);
#28168=VERTEX_POINT('',#97955);
#28169=VERTEX_POINT('',#97957);
#28170=VERTEX_POINT('',#97961);
#28171=VERTEX_POINT('',#97965);
#28172=VERTEX_POINT('',#97967);
#28173=VERTEX_POINT('',#97971);
#28174=VERTEX_POINT('',#97975);
#28175=VERTEX_POINT('',#97977);
#28176=VERTEX_POINT('',#97981);
#28177=VERTEX_POINT('',#97985);
#28178=VERTEX_POINT('',#97987);
#28179=VERTEX_POINT('',#97991);
#28180=VERTEX_POINT('',#97995);
#28181=VERTEX_POINT('',#97997);
#28182=VERTEX_POINT('',#98001);
#28183=VERTEX_POINT('',#98005);
#28184=VERTEX_POINT('',#98007);
#28185=VERTEX_POINT('',#98011);
#28186=VERTEX_POINT('',#98015);
#28187=VERTEX_POINT('',#98017);
#28188=VERTEX_POINT('',#98021);
#28189=VERTEX_POINT('',#98024);
#28190=VERTEX_POINT('',#98028);
#28191=VERTEX_POINT('',#98030);
#28192=VERTEX_POINT('',#98034);
#28193=VERTEX_POINT('',#98038);
#28194=VERTEX_POINT('',#98040);
#28195=VERTEX_POINT('',#98044);
#28196=VERTEX_POINT('',#98048);
#28197=VERTEX_POINT('',#98050);
#28198=VERTEX_POINT('',#98054);
#28199=VERTEX_POINT('',#98058);
#28200=VERTEX_POINT('',#98060);
#28201=VERTEX_POINT('',#98064);
#28202=VERTEX_POINT('',#98068);
#28203=VERTEX_POINT('',#98070);
#28204=VERTEX_POINT('',#98074);
#28205=VERTEX_POINT('',#98078);
#28206=VERTEX_POINT('',#98080);
#28207=VERTEX_POINT('',#98084);
#28208=VERTEX_POINT('',#98088);
#28209=VERTEX_POINT('',#98090);
#28210=VERTEX_POINT('',#98094);
#28211=VERTEX_POINT('',#98098);
#28212=VERTEX_POINT('',#98100);
#28213=VERTEX_POINT('',#98104);
#28214=VERTEX_POINT('',#98108);
#28215=VERTEX_POINT('',#98110);
#28216=VERTEX_POINT('',#98114);
#28217=VERTEX_POINT('',#98118);
#28218=VERTEX_POINT('',#98120);
#28219=VERTEX_POINT('',#98124);
#28220=VERTEX_POINT('',#98128);
#28221=VERTEX_POINT('',#98130);
#28222=VERTEX_POINT('',#98134);
#28223=VERTEX_POINT('',#98138);
#28224=VERTEX_POINT('',#98140);
#28225=VERTEX_POINT('',#98144);
#28226=VERTEX_POINT('',#98148);
#28227=VERTEX_POINT('',#98150);
#28228=VERTEX_POINT('',#98154);
#28229=VERTEX_POINT('',#98158);
#28230=VERTEX_POINT('',#98160);
#28231=VERTEX_POINT('',#98164);
#28232=VERTEX_POINT('',#98168);
#28233=VERTEX_POINT('',#98170);
#28234=VERTEX_POINT('',#98174);
#28235=VERTEX_POINT('',#98178);
#28236=VERTEX_POINT('',#98180);
#28237=VERTEX_POINT('',#98184);
#28238=VERTEX_POINT('',#98188);
#28239=VERTEX_POINT('',#98190);
#28240=VERTEX_POINT('',#98194);
#28241=VERTEX_POINT('',#98198);
#28242=VERTEX_POINT('',#98200);
#28243=VERTEX_POINT('',#98204);
#28244=VERTEX_POINT('',#98208);
#28245=VERTEX_POINT('',#98210);
#28246=VERTEX_POINT('',#98214);
#28247=VERTEX_POINT('',#98218);
#28248=VERTEX_POINT('',#98220);
#28249=VERTEX_POINT('',#98224);
#28250=VERTEX_POINT('',#98230);
#28251=VERTEX_POINT('',#98234);
#28252=VERTEX_POINT('',#98238);
#28253=VERTEX_POINT('',#98240);
#28254=VERTEX_POINT('',#98250);
#28255=VERTEX_POINT('',#98254);
#28256=VERTEX_POINT('',#98256);
#28257=VERTEX_POINT('',#98258);
#28258=VERTEX_POINT('',#98262);
#28259=VERTEX_POINT('',#98264);
#28260=VERTEX_POINT('',#98268);
#28261=VERTEX_POINT('',#98272);
#28262=VERTEX_POINT('',#98274);
#28263=VERTEX_POINT('',#98278);
#28264=VERTEX_POINT('',#98282);
#28265=VERTEX_POINT('',#98284);
#28266=VERTEX_POINT('',#98288);
#28267=VERTEX_POINT('',#98292);
#28268=VERTEX_POINT('',#98294);
#28269=VERTEX_POINT('',#98298);
#28270=VERTEX_POINT('',#98302);
#28271=VERTEX_POINT('',#98304);
#28272=VERTEX_POINT('',#98308);
#28273=VERTEX_POINT('',#98312);
#28274=VERTEX_POINT('',#98314);
#28275=VERTEX_POINT('',#98318);
#28276=VERTEX_POINT('',#98322);
#28277=VERTEX_POINT('',#98324);
#28278=VERTEX_POINT('',#98328);
#28279=VERTEX_POINT('',#98332);
#28280=VERTEX_POINT('',#98334);
#28281=VERTEX_POINT('',#98338);
#28282=VERTEX_POINT('',#98342);
#28283=VERTEX_POINT('',#98344);
#28284=VERTEX_POINT('',#98348);
#28285=VERTEX_POINT('',#98352);
#28286=VERTEX_POINT('',#98354);
#28287=VERTEX_POINT('',#98358);
#28288=VERTEX_POINT('',#98362);
#28289=VERTEX_POINT('',#98364);
#28290=VERTEX_POINT('',#98368);
#28291=VERTEX_POINT('',#98372);
#28292=VERTEX_POINT('',#98374);
#28293=VERTEX_POINT('',#98378);
#28294=VERTEX_POINT('',#98382);
#28295=VERTEX_POINT('',#98384);
#28296=VERTEX_POINT('',#98388);
#28297=VERTEX_POINT('',#98392);
#28298=VERTEX_POINT('',#98394);
#28299=VERTEX_POINT('',#98398);
#28300=VERTEX_POINT('',#98402);
#28301=VERTEX_POINT('',#98404);
#28302=VERTEX_POINT('',#98408);
#28303=VERTEX_POINT('',#98412);
#28304=VERTEX_POINT('',#98414);
#28305=VERTEX_POINT('',#98418);
#28306=VERTEX_POINT('',#98422);
#28307=VERTEX_POINT('',#98424);
#28308=VERTEX_POINT('',#98431);
#28309=VERTEX_POINT('',#98435);
#28310=VERTEX_POINT('',#98439);
#28311=VERTEX_POINT('',#98441);
#28312=VERTEX_POINT('',#98445);
#28313=VERTEX_POINT('',#98449);
#28314=VERTEX_POINT('',#98451);
#28315=VERTEX_POINT('',#98455);
#28316=VERTEX_POINT('',#98459);
#28317=VERTEX_POINT('',#98461);
#28318=VERTEX_POINT('',#98465);
#28319=VERTEX_POINT('',#98469);
#28320=VERTEX_POINT('',#98471);
#28321=VERTEX_POINT('',#98475);
#28322=VERTEX_POINT('',#98479);
#28323=VERTEX_POINT('',#98481);
#28324=VERTEX_POINT('',#98485);
#28325=VERTEX_POINT('',#98489);
#28326=VERTEX_POINT('',#98491);
#28327=VERTEX_POINT('',#98495);
#28328=VERTEX_POINT('',#98499);
#28329=VERTEX_POINT('',#98501);
#28330=VERTEX_POINT('',#98505);
#28331=VERTEX_POINT('',#98509);
#28332=VERTEX_POINT('',#98511);
#28333=VERTEX_POINT('',#98515);
#28334=VERTEX_POINT('',#98519);
#28335=VERTEX_POINT('',#98521);
#28336=VERTEX_POINT('',#98525);
#28337=VERTEX_POINT('',#98529);
#28338=VERTEX_POINT('',#98531);
#28339=VERTEX_POINT('',#98535);
#28340=VERTEX_POINT('',#98539);
#28341=VERTEX_POINT('',#98541);
#28342=VERTEX_POINT('',#98545);
#28343=VERTEX_POINT('',#98549);
#28344=VERTEX_POINT('',#98551);
#28345=VERTEX_POINT('',#98555);
#28346=VERTEX_POINT('',#98559);
#28347=VERTEX_POINT('',#98561);
#28348=VERTEX_POINT('',#98565);
#28349=VERTEX_POINT('',#98569);
#28350=VERTEX_POINT('',#98571);
#28351=VERTEX_POINT('',#98575);
#28352=VERTEX_POINT('',#98579);
#28353=VERTEX_POINT('',#98581);
#28354=VERTEX_POINT('',#98585);
#28355=VERTEX_POINT('',#98589);
#28356=VERTEX_POINT('',#98591);
#28357=VERTEX_POINT('',#98595);
#28358=VERTEX_POINT('',#98599);
#28359=VERTEX_POINT('',#98601);
#28360=VERTEX_POINT('',#98605);
#28361=VERTEX_POINT('',#98609);
#28362=VERTEX_POINT('',#98611);
#28363=VERTEX_POINT('',#98615);
#28364=VERTEX_POINT('',#98619);
#28365=VERTEX_POINT('',#98621);
#28366=VERTEX_POINT('',#98625);
#28367=VERTEX_POINT('',#98629);
#28368=VERTEX_POINT('',#98859);
#28369=VERTEX_POINT('',#98861);
#28370=VERTEX_POINT('',#98865);
#28371=VERTEX_POINT('',#98868);
#28372=VERTEX_POINT('',#98872);
#28373=VERTEX_POINT('',#98876);
#28374=VERTEX_POINT('',#98880);
#28375=VERTEX_POINT('',#98883);
#28376=VERTEX_POINT('',#98887);
#28377=VERTEX_POINT('',#98893);
#28378=VERTEX_POINT('',#98896);
#28379=VERTEX_POINT('',#98901);
#28380=VERTEX_POINT('',#98902);
#35636=EDGE_CURVE('',#28118,#28119,#14496,.T.);
#35637=EDGE_CURVE('',#28120,#28118,#1137,.T.);
#35638=EDGE_CURVE('',#28119,#28120,#1138,.T.);
#35639=EDGE_CURVE('',#28121,#28122,#24345,.T.);
#35640=EDGE_CURVE('',#28123,#28121,#24346,.T.);
#35641=EDGE_CURVE('',#28122,#28123,#24347,.T.);
#35642=EDGE_CURVE('',#28122,#28120,#14497,.T.);
#35643=EDGE_CURVE('',#28124,#28118,#24348,.T.);
#35644=EDGE_CURVE('',#28124,#28125,#1139,.T.);
#35645=EDGE_CURVE('',#28119,#28125,#24349,.T.);
#35646=EDGE_CURVE('',#28125,#28124,#14498,.T.);
#35647=EDGE_CURVE('',#28126,#28127,#211,.T.);
#35648=EDGE_CURVE('',#28126,#28128,#14499,.T.);
#35649=EDGE_CURVE('',#28129,#28128,#212,.T.);
#35650=EDGE_CURVE('',#28127,#28129,#14500,.T.);
#35651=EDGE_CURVE('',#28130,#28126,#213,.T.);
#35652=EDGE_CURVE('',#28131,#28130,#14501,.T.);
#35653=EDGE_CURVE('',#28128,#28131,#214,.T.);
#35654=EDGE_CURVE('',#28132,#28131,#1140,.T.);
#35655=EDGE_CURVE('',#28132,#28133,#215,.T.);
#35656=EDGE_CURVE('',#28133,#28134,#216,.T.);
#35657=EDGE_CURVE('',#28135,#28134,#1141,.T.);
#35658=EDGE_CURVE('',#28135,#28136,#217,.T.);
#35659=EDGE_CURVE('',#28136,#28137,#218,.T.);
#35660=EDGE_CURVE('',#28138,#28137,#1142,.T.);
#35661=EDGE_CURVE('',#28138,#28139,#219,.T.);
#35662=EDGE_CURVE('',#28139,#28140,#220,.T.);
#35663=EDGE_CURVE('',#28141,#28140,#1143,.T.);
#35664=EDGE_CURVE('',#28141,#28142,#221,.T.);
#35665=EDGE_CURVE('',#28142,#28143,#222,.T.);
#35666=EDGE_CURVE('',#28144,#28143,#1144,.T.);
#35667=EDGE_CURVE('',#28144,#28145,#223,.T.);
#35668=EDGE_CURVE('',#28145,#28146,#224,.T.);
#35669=EDGE_CURVE('',#28147,#28146,#1145,.T.);
#35670=EDGE_CURVE('',#28147,#28148,#225,.T.);
#35671=EDGE_CURVE('',#28148,#28149,#226,.T.);
#35672=EDGE_CURVE('',#28150,#28149,#1146,.T.);
#35673=EDGE_CURVE('',#28150,#28151,#227,.T.);
#35674=EDGE_CURVE('',#28151,#28152,#228,.T.);
#35675=EDGE_CURVE('',#28153,#28152,#1147,.T.);
#35676=EDGE_CURVE('',#28153,#28154,#229,.T.);
#35677=EDGE_CURVE('',#28154,#28155,#230,.T.);
#35678=EDGE_CURVE('',#28156,#28155,#1148,.T.);
#35679=EDGE_CURVE('',#28156,#28157,#231,.T.);
#35680=EDGE_CURVE('',#28157,#28158,#232,.T.);
#35681=EDGE_CURVE('',#28159,#28158,#1149,.T.);
#35682=EDGE_CURVE('',#28159,#28160,#233,.T.);
#35683=EDGE_CURVE('',#28160,#28161,#234,.T.);
#35684=EDGE_CURVE('',#28162,#28161,#1150,.T.);
#35685=EDGE_CURVE('',#28162,#28163,#235,.T.);
#35686=EDGE_CURVE('',#28163,#28164,#236,.T.);
#35687=EDGE_CURVE('',#28165,#28164,#1151,.T.);
#35688=EDGE_CURVE('',#28165,#28166,#237,.T.);
#35689=EDGE_CURVE('',#28166,#28167,#238,.T.);
#35690=EDGE_CURVE('',#28168,#28167,#1152,.T.);
#35691=EDGE_CURVE('',#28168,#28169,#239,.T.);
#35692=EDGE_CURVE('',#28169,#28170,#240,.T.);
#35693=EDGE_CURVE('',#28171,#28170,#1153,.T.);
#35694=EDGE_CURVE('',#28171,#28172,#241,.T.);
#35695=EDGE_CURVE('',#28172,#28173,#242,.T.);
#35696=EDGE_CURVE('',#28174,#28173,#1154,.T.);
#35697=EDGE_CURVE('',#28174,#28175,#243,.T.);
#35698=EDGE_CURVE('',#28175,#28176,#244,.T.);
#35699=EDGE_CURVE('',#28177,#28176,#1155,.T.);
#35700=EDGE_CURVE('',#28177,#28178,#245,.T.);
#35701=EDGE_CURVE('',#28178,#28179,#246,.T.);
#35702=EDGE_CURVE('',#28180,#28179,#1156,.T.);
#35703=EDGE_CURVE('',#28180,#28181,#247,.T.);
#35704=EDGE_CURVE('',#28181,#28182,#248,.T.);
#35705=EDGE_CURVE('',#28183,#28182,#1157,.T.);
#35706=EDGE_CURVE('',#28183,#28184,#249,.T.);
#35707=EDGE_CURVE('',#28184,#28185,#250,.T.);
#35708=EDGE_CURVE('',#28186,#28185,#1158,.T.);
#35709=EDGE_CURVE('',#28186,#28187,#251,.T.);
#35710=EDGE_CURVE('',#28187,#28188,#14502,.T.);
#35711=EDGE_CURVE('',#28188,#28188,#1159,.T.);
#35712=EDGE_CURVE('',#28187,#28189,#252,.T.);
#35713=EDGE_CURVE('',#28190,#28189,#1160,.T.);
#35714=EDGE_CURVE('',#28190,#28191,#253,.T.);
#35715=EDGE_CURVE('',#28191,#28192,#254,.T.);
#35716=EDGE_CURVE('',#28193,#28192,#1161,.T.);
#35717=EDGE_CURVE('',#28193,#28194,#255,.T.);
#35718=EDGE_CURVE('',#28194,#28195,#256,.T.);
#35719=EDGE_CURVE('',#28196,#28195,#1162,.T.);
#35720=EDGE_CURVE('',#28196,#28197,#257,.T.);
#35721=EDGE_CURVE('',#28197,#28198,#258,.T.);
#35722=EDGE_CURVE('',#28199,#28198,#1163,.T.);
#35723=EDGE_CURVE('',#28199,#28200,#259,.T.);
#35724=EDGE_CURVE('',#28200,#28201,#260,.T.);
#35725=EDGE_CURVE('',#28202,#28201,#1164,.T.);
#35726=EDGE_CURVE('',#28202,#28203,#261,.T.);
#35727=EDGE_CURVE('',#28203,#28204,#262,.T.);
#35728=EDGE_CURVE('',#28205,#28204,#1165,.T.);
#35729=EDGE_CURVE('',#28205,#28206,#263,.T.);
#35730=EDGE_CURVE('',#28206,#28207,#264,.T.);
#35731=EDGE_CURVE('',#28208,#28207,#1166,.T.);
#35732=EDGE_CURVE('',#28208,#28209,#265,.T.);
#35733=EDGE_CURVE('',#28209,#28210,#266,.T.);
#35734=EDGE_CURVE('',#28211,#28210,#1167,.T.);
#35735=EDGE_CURVE('',#28211,#28212,#267,.T.);
#35736=EDGE_CURVE('',#28212,#28213,#268,.T.);
#35737=EDGE_CURVE('',#28214,#28213,#1168,.T.);
#35738=EDGE_CURVE('',#28214,#28215,#269,.T.);
#35739=EDGE_CURVE('',#28215,#28216,#270,.T.);
#35740=EDGE_CURVE('',#28217,#28216,#1169,.T.);
#35741=EDGE_CURVE('',#28217,#28218,#271,.T.);
#35742=EDGE_CURVE('',#28218,#28219,#272,.T.);
#35743=EDGE_CURVE('',#28220,#28219,#1170,.T.);
#35744=EDGE_CURVE('',#28220,#28221,#273,.T.);
#35745=EDGE_CURVE('',#28221,#28222,#274,.T.);
#35746=EDGE_CURVE('',#28223,#28222,#1171,.T.);
#35747=EDGE_CURVE('',#28223,#28224,#275,.T.);
#35748=EDGE_CURVE('',#28224,#28225,#276,.T.);
#35749=EDGE_CURVE('',#28226,#28225,#1172,.T.);
#35750=EDGE_CURVE('',#28226,#28227,#277,.T.);
#35751=EDGE_CURVE('',#28227,#28228,#278,.T.);
#35752=EDGE_CURVE('',#28229,#28228,#1173,.T.);
#35753=EDGE_CURVE('',#28229,#28230,#279,.T.);
#35754=EDGE_CURVE('',#28230,#28231,#280,.T.);
#35755=EDGE_CURVE('',#28232,#28231,#1174,.T.);
#35756=EDGE_CURVE('',#28232,#28233,#281,.T.);
#35757=EDGE_CURVE('',#28233,#28234,#282,.T.);
#35758=EDGE_CURVE('',#28235,#28234,#1175,.T.);
#35759=EDGE_CURVE('',#28235,#28236,#283,.T.);
#35760=EDGE_CURVE('',#28236,#28237,#284,.T.);
#35761=EDGE_CURVE('',#28238,#28237,#1176,.T.);
#35762=EDGE_CURVE('',#28238,#28239,#285,.T.);
#35763=EDGE_CURVE('',#28239,#28240,#286,.T.);
#35764=EDGE_CURVE('',#28241,#28240,#1177,.T.);
#35765=EDGE_CURVE('',#28241,#28242,#287,.T.);
#35766=EDGE_CURVE('',#28242,#28243,#288,.T.);
#35767=EDGE_CURVE('',#28244,#28243,#1178,.T.);
#35768=EDGE_CURVE('',#28244,#28245,#289,.T.);
#35769=EDGE_CURVE('',#28245,#28246,#290,.T.);
#35770=EDGE_CURVE('',#28247,#28246,#1179,.T.);
#35771=EDGE_CURVE('',#28247,#28248,#291,.T.);
#35772=EDGE_CURVE('',#28248,#28249,#292,.T.);
#35773=EDGE_CURVE('',#28129,#28249,#1180,.T.);
#35774=EDGE_CURVE('',#28250,#28130,#1181,.T.);
#35775=EDGE_CURVE('',#28250,#28132,#14503,.T.);
#35776=EDGE_CURVE('',#28249,#28251,#14504,.T.);
#35777=EDGE_CURVE('',#28127,#28251,#1182,.T.);
#35778=EDGE_CURVE('',#28252,#28133,#14505,.T.);
#35779=EDGE_CURVE('',#28253,#28252,#293,.T.);
#35780=EDGE_CURVE('',#28134,#28253,#14506,.T.);
#35781=EDGE_CURVE('',#28252,#28250,#294,.T.);
#35782=EDGE_CURVE('',#28254,#28253,#1183,.T.);
#35783=EDGE_CURVE('',#28254,#28135,#14507,.T.);
#35784=EDGE_CURVE('',#28255,#28255,#1184,.T.);
#35785=EDGE_CURVE('',#28255,#28256,#14508,.T.);
#35786=EDGE_CURVE('',#28256,#28257,#295,.T.);
#35787=EDGE_CURVE('',#28257,#28258,#1185,.T.);
#35788=EDGE_CURVE('',#28258,#28259,#296,.T.);
#35789=EDGE_CURVE('',#28259,#28260,#297,.T.);
#35790=EDGE_CURVE('',#28260,#28261,#1186,.T.);
#35791=EDGE_CURVE('',#28261,#28262,#298,.T.);
#35792=EDGE_CURVE('',#28262,#28263,#299,.T.);
#35793=EDGE_CURVE('',#28263,#28264,#1187,.T.);
#35794=EDGE_CURVE('',#28264,#28265,#300,.T.);
#35795=EDGE_CURVE('',#28265,#28266,#301,.T.);
#35796=EDGE_CURVE('',#28266,#28267,#1188,.T.);
#35797=EDGE_CURVE('',#28267,#28268,#302,.T.);
#35798=EDGE_CURVE('',#28268,#28269,#303,.T.);
#35799=EDGE_CURVE('',#28269,#28270,#1189,.T.);
#35800=EDGE_CURVE('',#28270,#28271,#304,.T.);
#35801=EDGE_CURVE('',#28271,#28272,#305,.T.);
#35802=EDGE_CURVE('',#28272,#28273,#1190,.T.);
#35803=EDGE_CURVE('',#28273,#28274,#306,.T.);
#35804=EDGE_CURVE('',#28274,#28275,#307,.T.);
#35805=EDGE_CURVE('',#28275,#28276,#1191,.T.);
#35806=EDGE_CURVE('',#28276,#28277,#308,.T.);
#35807=EDGE_CURVE('',#28277,#28278,#309,.T.);
#35808=EDGE_CURVE('',#28278,#28279,#1192,.T.);
#35809=EDGE_CURVE('',#28279,#28280,#310,.T.);
#35810=EDGE_CURVE('',#28280,#28281,#311,.T.);
#35811=EDGE_CURVE('',#28281,#28282,#1193,.T.);
#35812=EDGE_CURVE('',#28282,#28283,#312,.T.);
#35813=EDGE_CURVE('',#28283,#28284,#313,.T.);
#35814=EDGE_CURVE('',#28284,#28285,#1194,.T.);
#35815=EDGE_CURVE('',#28285,#28286,#314,.T.);
#35816=EDGE_CURVE('',#28286,#28287,#315,.T.);
#35817=EDGE_CURVE('',#28287,#28288,#1195,.T.);
#35818=EDGE_CURVE('',#28288,#28289,#316,.T.);
#35819=EDGE_CURVE('',#28289,#28290,#317,.T.);
#35820=EDGE_CURVE('',#28290,#28291,#1196,.T.);
#35821=EDGE_CURVE('',#28291,#28292,#318,.T.);
#35822=EDGE_CURVE('',#28292,#28293,#319,.T.);
#35823=EDGE_CURVE('',#28293,#28294,#1197,.T.);
#35824=EDGE_CURVE('',#28294,#28295,#320,.T.);
#35825=EDGE_CURVE('',#28295,#28296,#321,.T.);
#35826=EDGE_CURVE('',#28296,#28297,#1198,.T.);
#35827=EDGE_CURVE('',#28297,#28298,#322,.T.);
#35828=EDGE_CURVE('',#28298,#28299,#323,.T.);
#35829=EDGE_CURVE('',#28299,#28300,#1199,.T.);
#35830=EDGE_CURVE('',#28300,#28301,#324,.T.);
#35831=EDGE_CURVE('',#28301,#28302,#325,.T.);
#35832=EDGE_CURVE('',#28302,#28303,#1200,.T.);
#35833=EDGE_CURVE('',#28303,#28304,#326,.T.);
#35834=EDGE_CURVE('',#28304,#28305,#327,.T.);
#35835=EDGE_CURVE('',#28305,#28306,#1201,.T.);
#35836=EDGE_CURVE('',#28306,#28307,#328,.T.);
#35837=EDGE_CURVE('',#28307,#28254,#329,.T.);
#35838=EDGE_CURVE('',#28251,#28308,#330,.T.);
#35839=EDGE_CURVE('',#28308,#28309,#331,.T.);
#35840=EDGE_CURVE('',#28309,#28310,#1202,.T.);
#35841=EDGE_CURVE('',#28310,#28311,#332,.T.);
#35842=EDGE_CURVE('',#28311,#28312,#333,.T.);
#35843=EDGE_CURVE('',#28312,#28313,#1203,.T.);
#35844=EDGE_CURVE('',#28313,#28314,#334,.T.);
#35845=EDGE_CURVE('',#28314,#28315,#335,.T.);
#35846=EDGE_CURVE('',#28315,#28316,#1204,.T.);
#35847=EDGE_CURVE('',#28316,#28317,#336,.T.);
#35848=EDGE_CURVE('',#28317,#28318,#337,.T.);
#35849=EDGE_CURVE('',#28318,#28319,#1205,.T.);
#35850=EDGE_CURVE('',#28319,#28320,#338,.T.);
#35851=EDGE_CURVE('',#28320,#28321,#339,.T.);
#35852=EDGE_CURVE('',#28321,#28322,#1206,.T.);
#35853=EDGE_CURVE('',#28322,#28323,#340,.T.);
#35854=EDGE_CURVE('',#28323,#28324,#341,.T.);
#35855=EDGE_CURVE('',#28324,#28325,#1207,.T.);
#35856=EDGE_CURVE('',#28325,#28326,#342,.T.);
#35857=EDGE_CURVE('',#28326,#28327,#343,.T.);
#35858=EDGE_CURVE('',#28327,#28328,#1208,.T.);
#35859=EDGE_CURVE('',#28328,#28329,#344,.T.);
#35860=EDGE_CURVE('',#28329,#28330,#345,.T.);
#35861=EDGE_CURVE('',#28330,#28331,#1209,.T.);
#35862=EDGE_CURVE('',#28331,#28332,#346,.T.);
#35863=EDGE_CURVE('',#28332,#28333,#347,.T.);
#35864=EDGE_CURVE('',#28333,#28334,#1210,.T.);
#35865=EDGE_CURVE('',#28334,#28335,#348,.T.);
#35866=EDGE_CURVE('',#28335,#28336,#349,.T.);
#35867=EDGE_CURVE('',#28336,#28337,#1211,.T.);
#35868=EDGE_CURVE('',#28337,#28338,#350,.T.);
#35869=EDGE_CURVE('',#28338,#28339,#351,.T.);
#35870=EDGE_CURVE('',#28339,#28340,#1212,.T.);
#35871=EDGE_CURVE('',#28340,#28341,#352,.T.);
#35872=EDGE_CURVE('',#28341,#28342,#353,.T.);
#35873=EDGE_CURVE('',#28342,#28343,#1213,.T.);
#35874=EDGE_CURVE('',#28343,#28344,#354,.T.);
#35875=EDGE_CURVE('',#28344,#28345,#355,.T.);
#35876=EDGE_CURVE('',#28345,#28346,#1214,.T.);
#35877=EDGE_CURVE('',#28346,#28347,#356,.T.);
#35878=EDGE_CURVE('',#28347,#28348,#357,.T.);
#35879=EDGE_CURVE('',#28348,#28349,#1215,.T.);
#35880=EDGE_CURVE('',#28349,#28350,#358,.T.);
#35881=EDGE_CURVE('',#28350,#28351,#359,.T.);
#35882=EDGE_CURVE('',#28351,#28352,#1216,.T.);
#35883=EDGE_CURVE('',#28352,#28353,#360,.T.);
#35884=EDGE_CURVE('',#28353,#28354,#361,.T.);
#35885=EDGE_CURVE('',#28354,#28355,#1217,.T.);
#35886=EDGE_CURVE('',#28355,#28356,#362,.T.);
#35887=EDGE_CURVE('',#28356,#28357,#363,.T.);
#35888=EDGE_CURVE('',#28357,#28358,#1218,.T.);
#35889=EDGE_CURVE('',#28358,#28359,#364,.T.);
#35890=EDGE_CURVE('',#28359,#28360,#365,.T.);
#35891=EDGE_CURVE('',#28360,#28361,#1219,.T.);
#35892=EDGE_CURVE('',#28361,#28362,#366,.T.);
#35893=EDGE_CURVE('',#28362,#28363,#367,.T.);
#35894=EDGE_CURVE('',#28363,#28364,#1220,.T.);
#35895=EDGE_CURVE('',#28364,#28365,#368,.T.);
#35896=EDGE_CURVE('',#28365,#28366,#369,.T.);
#35897=EDGE_CURVE('',#28366,#28367,#1221,.T.);
#35898=EDGE_CURVE('',#28367,#28256,#370,.T.);
#35899=EDGE_CURVE('',#28307,#28136,#14509,.T.);
#35900=EDGE_CURVE('',#28137,#28306,#14510,.T.);
#35901=EDGE_CURVE('',#28304,#28139,#14511,.T.);
#35902=EDGE_CURVE('',#28305,#28138,#14512,.T.);
#35903=EDGE_CURVE('',#28140,#28303,#14513,.T.);
#35904=EDGE_CURVE('',#28302,#28141,#14514,.T.);
#35905=EDGE_CURVE('',#28301,#28142,#14515,.T.);
#35906=EDGE_CURVE('',#28143,#28300,#14516,.T.);
#35907=EDGE_CURVE('',#28299,#28144,#14517,.T.);
#35908=EDGE_CURVE('',#28298,#28145,#14518,.T.);
#35909=EDGE_CURVE('',#28146,#28297,#14519,.T.);
#35910=EDGE_CURVE('',#28295,#28148,#14520,.T.);
#35911=EDGE_CURVE('',#28296,#28147,#14521,.T.);
#35912=EDGE_CURVE('',#28149,#28294,#14522,.T.);
#35913=EDGE_CURVE('',#28293,#28150,#14523,.T.);
#35914=EDGE_CURVE('',#28292,#28151,#14524,.T.);
#35915=EDGE_CURVE('',#28152,#28291,#14525,.T.);
#35916=EDGE_CURVE('',#28290,#28153,#14526,.T.);
#35917=EDGE_CURVE('',#28289,#28154,#14527,.T.);
#35918=EDGE_CURVE('',#28155,#28288,#14528,.T.);
#35919=EDGE_CURVE('',#28286,#28157,#14529,.T.);
#35920=EDGE_CURVE('',#28287,#28156,#14530,.T.);
#35921=EDGE_CURVE('',#28158,#28285,#14531,.T.);
#35922=EDGE_CURVE('',#28284,#28159,#14532,.T.);
#35923=EDGE_CURVE('',#28283,#28160,#14533,.T.);
#35924=EDGE_CURVE('',#28161,#28282,#14534,.T.);
#35925=EDGE_CURVE('',#28281,#28162,#14535,.T.);
#35926=EDGE_CURVE('',#28280,#28163,#14536,.T.);
#35927=EDGE_CURVE('',#28164,#28279,#14537,.T.);
#35928=EDGE_CURVE('',#28277,#28166,#14538,.T.);
#35929=EDGE_CURVE('',#28278,#28165,#14539,.T.);
#35930=EDGE_CURVE('',#28167,#28276,#14540,.T.);
#35931=EDGE_CURVE('',#28275,#28168,#14541,.T.);
#35932=EDGE_CURVE('',#28274,#28169,#14542,.T.);
#35933=EDGE_CURVE('',#28170,#28273,#14543,.T.);
#35934=EDGE_CURVE('',#28272,#28171,#14544,.T.);
#35935=EDGE_CURVE('',#28271,#28172,#14545,.T.);
#35936=EDGE_CURVE('',#28173,#28270,#14546,.T.);
#35937=EDGE_CURVE('',#28268,#28175,#14547,.T.);
#35938=EDGE_CURVE('',#28269,#28174,#14548,.T.);
#35939=EDGE_CURVE('',#28176,#28267,#14549,.T.);
#35940=EDGE_CURVE('',#28266,#28177,#14550,.T.);
#35941=EDGE_CURVE('',#28265,#28178,#14551,.T.);
#35942=EDGE_CURVE('',#28179,#28264,#14552,.T.);
#35943=EDGE_CURVE('',#28263,#28180,#14553,.T.);
#35944=EDGE_CURVE('',#28262,#28181,#14554,.T.);
#35945=EDGE_CURVE('',#28182,#28261,#14555,.T.);
#35946=EDGE_CURVE('',#28259,#28184,#14556,.T.);
#35947=EDGE_CURVE('',#28260,#28183,#14557,.T.);
#35948=EDGE_CURVE('',#28185,#28258,#14558,.T.);
#35949=EDGE_CURVE('',#28257,#28186,#14559,.T.);
#35950=EDGE_CURVE('',#28256,#28187,#14560,.T.);
#35951=EDGE_CURVE('',#28189,#28367,#14561,.T.);
#35952=EDGE_CURVE('',#28366,#28190,#14562,.T.);
#35953=EDGE_CURVE('',#28365,#28191,#14563,.T.);
#35954=EDGE_CURVE('',#28192,#28364,#14564,.T.);
#35955=EDGE_CURVE('',#28362,#28194,#14565,.T.);
#35956=EDGE_CURVE('',#28363,#28193,#14566,.T.);
#35957=EDGE_CURVE('',#28195,#28361,#14567,.T.);
#35958=EDGE_CURVE('',#28360,#28196,#14568,.T.);
#35959=EDGE_CURVE('',#28359,#28197,#14569,.T.);
#35960=EDGE_CURVE('',#28198,#28358,#14570,.T.);
#35961=EDGE_CURVE('',#28357,#28199,#14571,.T.);
#35962=EDGE_CURVE('',#28356,#28200,#14572,.T.);
#35963=EDGE_CURVE('',#28201,#28355,#14573,.T.);
#35964=EDGE_CURVE('',#28353,#28203,#14574,.T.);
#35965=EDGE_CURVE('',#28354,#28202,#14575,.T.);
#35966=EDGE_CURVE('',#28204,#28352,#14576,.T.);
#35967=EDGE_CURVE('',#28351,#28205,#14577,.T.);
#35968=EDGE_CURVE('',#28350,#28206,#14578,.T.);
#35969=EDGE_CURVE('',#28207,#28349,#14579,.T.);
#35970=EDGE_CURVE('',#28348,#28208,#14580,.T.);
#35971=EDGE_CURVE('',#28347,#28209,#14581,.T.);
#35972=EDGE_CURVE('',#28210,#28346,#14582,.T.);
#35973=EDGE_CURVE('',#28344,#28212,#14583,.T.);
#35974=EDGE_CURVE('',#28345,#28211,#14584,.T.);
#35975=EDGE_CURVE('',#28213,#28343,#14585,.T.);
#35976=EDGE_CURVE('',#28342,#28214,#14586,.T.);
#35977=EDGE_CURVE('',#28341,#28215,#14587,.T.);
#35978=EDGE_CURVE('',#28216,#28340,#14588,.T.);
#35979=EDGE_CURVE('',#28339,#28217,#14589,.T.);
#35980=EDGE_CURVE('',#28338,#28218,#14590,.T.);
#35981=EDGE_CURVE('',#28219,#28337,#14591,.T.);
#35982=EDGE_CURVE('',#28335,#28221,#14592,.T.);
#35983=EDGE_CURVE('',#28336,#28220,#14593,.T.);
#35984=EDGE_CURVE('',#28222,#28334,#14594,.T.);
#35985=EDGE_CURVE('',#28333,#28223,#14595,.T.);
#35986=EDGE_CURVE('',#28332,#28224,#14596,.T.);
#35987=EDGE_CURVE('',#28225,#28331,#14597,.T.);
#35988=EDGE_CURVE('',#28330,#28226,#14598,.T.);
#35989=EDGE_CURVE('',#28329,#28227,#14599,.T.);
#35990=EDGE_CURVE('',#28228,#28328,#14600,.T.);
#35991=EDGE_CURVE('',#28326,#28230,#14601,.T.);
#35992=EDGE_CURVE('',#28327,#28229,#14602,.T.);
#35993=EDGE_CURVE('',#28231,#28325,#14603,.T.);
#35994=EDGE_CURVE('',#28324,#28232,#14604,.T.);
#35995=EDGE_CURVE('',#28323,#28233,#14605,.T.);
#35996=EDGE_CURVE('',#28234,#28322,#14606,.T.);
#35997=EDGE_CURVE('',#28321,#28235,#14607,.T.);
#35998=EDGE_CURVE('',#28320,#28236,#14608,.T.);
#35999=EDGE_CURVE('',#28237,#28319,#14609,.T.);
#36000=EDGE_CURVE('',#28317,#28239,#14610,.T.);
#36001=EDGE_CURVE('',#28318,#28238,#14611,.T.);
#36002=EDGE_CURVE('',#28240,#28316,#14612,.T.);
#36003=EDGE_CURVE('',#28315,#28241,#14613,.T.);
#36004=EDGE_CURVE('',#28314,#28242,#14614,.T.);
#36005=EDGE_CURVE('',#28243,#28313,#14615,.T.);
#36006=EDGE_CURVE('',#28312,#28244,#14616,.T.);
#36007=EDGE_CURVE('',#28311,#28245,#14617,.T.);
#36008=EDGE_CURVE('',#28246,#28310,#14618,.T.);
#36009=EDGE_CURVE('',#28308,#28248,#14619,.T.);
#36010=EDGE_CURVE('',#28309,#28247,#14620,.T.);
#36011=EDGE_CURVE('',#28368,#28368,#1222,.T.);
#36012=EDGE_CURVE('',#28368,#28369,#14621,.T.);
#36013=EDGE_CURVE('',#28369,#28369,#1223,.T.);
#36014=EDGE_CURVE('',#28370,#28370,#1224,.T.);
#36015=EDGE_CURVE('',#28371,#28371,#1225,.T.);
#36016=EDGE_CURVE('',#28371,#28370,#14622,.T.);
#36017=EDGE_CURVE('',#28372,#28372,#1226,.T.);
#36018=EDGE_CURVE('',#28372,#28371,#14623,.T.);
#36019=EDGE_CURVE('',#28373,#28373,#1227,.T.);
#36020=EDGE_CURVE('',#28373,#28372,#14624,.T.);
#36021=EDGE_CURVE('',#28374,#28374,#1228,.T.);
#36022=EDGE_CURVE('',#28375,#28375,#1229,.T.);
#36023=EDGE_CURVE('',#28375,#28374,#14625,.T.);
#36024=EDGE_CURVE('',#28376,#28376,#1230,.T.);
#36025=EDGE_CURVE('',#28376,#28375,#14626,.T.);
#36026=EDGE_CURVE('',#28377,#28377,#1231,.T.);
#36027=EDGE_CURVE('',#28377,#28378,#14627,.T.);
#36028=EDGE_CURVE('',#28378,#28378,#1232,.T.);
#36029=EDGE_CURVE('',#28379,#28380,#14628,.T.);
#36030=EDGE_CURVE('',#28380,#28380,#1233,.T.);
#36031=EDGE_CURVE('',#28380,#28368,#14629,.T.);
#49607=ORIENTED_EDGE('',*,*,#35636,.F.);
#49608=ORIENTED_EDGE('',*,*,#35637,.F.);
#49609=ORIENTED_EDGE('',*,*,#35638,.F.);
#49610=ORIENTED_EDGE('',*,*,#35639,.F.);
#49611=ORIENTED_EDGE('',*,*,#35640,.F.);
#49612=ORIENTED_EDGE('',*,*,#35641,.F.);
#49613=ORIENTED_EDGE('',*,*,#35642,.T.);
#49614=ORIENTED_EDGE('',*,*,#35637,.T.);
#49615=ORIENTED_EDGE('',*,*,#35643,.F.);
#49616=ORIENTED_EDGE('',*,*,#35644,.T.);
#49617=ORIENTED_EDGE('',*,*,#35645,.F.);
#49618=ORIENTED_EDGE('',*,*,#35638,.T.);
#49619=ORIENTED_EDGE('',*,*,#35642,.F.);
#49620=ORIENTED_EDGE('',*,*,#35646,.F.);
#49621=ORIENTED_EDGE('',*,*,#35644,.F.);
#49622=ORIENTED_EDGE('',*,*,#35647,.F.);
#49623=ORIENTED_EDGE('',*,*,#35648,.T.);
#49624=ORIENTED_EDGE('',*,*,#35649,.F.);
#49625=ORIENTED_EDGE('',*,*,#35650,.F.);
#49626=ORIENTED_EDGE('',*,*,#35651,.F.);
#49627=ORIENTED_EDGE('',*,*,#35652,.F.);
#49628=ORIENTED_EDGE('',*,*,#35653,.F.);
#49629=ORIENTED_EDGE('',*,*,#35648,.F.);
#49630=ORIENTED_EDGE('',*,*,#35649,.T.);
#49631=ORIENTED_EDGE('',*,*,#35653,.T.);
#49632=ORIENTED_EDGE('',*,*,#35654,.F.);
#49633=ORIENTED_EDGE('',*,*,#35655,.T.);
#49634=ORIENTED_EDGE('',*,*,#35656,.T.);
#49635=ORIENTED_EDGE('',*,*,#35657,.F.);
#49636=ORIENTED_EDGE('',*,*,#35658,.T.);
#49637=ORIENTED_EDGE('',*,*,#35659,.T.);
#49638=ORIENTED_EDGE('',*,*,#35660,.F.);
#49639=ORIENTED_EDGE('',*,*,#35661,.T.);
#49640=ORIENTED_EDGE('',*,*,#35662,.T.);
#49641=ORIENTED_EDGE('',*,*,#35663,.F.);
#49642=ORIENTED_EDGE('',*,*,#35664,.T.);
#49643=ORIENTED_EDGE('',*,*,#35665,.T.);
#49644=ORIENTED_EDGE('',*,*,#35666,.F.);
#49645=ORIENTED_EDGE('',*,*,#35667,.T.);
#49646=ORIENTED_EDGE('',*,*,#35668,.T.);
#49647=ORIENTED_EDGE('',*,*,#35669,.F.);
#49648=ORIENTED_EDGE('',*,*,#35670,.T.);
#49649=ORIENTED_EDGE('',*,*,#35671,.T.);
#49650=ORIENTED_EDGE('',*,*,#35672,.F.);
#49651=ORIENTED_EDGE('',*,*,#35673,.T.);
#49652=ORIENTED_EDGE('',*,*,#35674,.T.);
#49653=ORIENTED_EDGE('',*,*,#35675,.F.);
#49654=ORIENTED_EDGE('',*,*,#35676,.T.);
#49655=ORIENTED_EDGE('',*,*,#35677,.T.);
#49656=ORIENTED_EDGE('',*,*,#35678,.F.);
#49657=ORIENTED_EDGE('',*,*,#35679,.T.);
#49658=ORIENTED_EDGE('',*,*,#35680,.T.);
#49659=ORIENTED_EDGE('',*,*,#35681,.F.);
#49660=ORIENTED_EDGE('',*,*,#35682,.T.);
#49661=ORIENTED_EDGE('',*,*,#35683,.T.);
#49662=ORIENTED_EDGE('',*,*,#35684,.F.);
#49663=ORIENTED_EDGE('',*,*,#35685,.T.);
#49664=ORIENTED_EDGE('',*,*,#35686,.T.);
#49665=ORIENTED_EDGE('',*,*,#35687,.F.);
#49666=ORIENTED_EDGE('',*,*,#35688,.T.);
#49667=ORIENTED_EDGE('',*,*,#35689,.T.);
#49668=ORIENTED_EDGE('',*,*,#35690,.F.);
#49669=ORIENTED_EDGE('',*,*,#35691,.T.);
#49670=ORIENTED_EDGE('',*,*,#35692,.T.);
#49671=ORIENTED_EDGE('',*,*,#35693,.F.);
#49672=ORIENTED_EDGE('',*,*,#35694,.T.);
#49673=ORIENTED_EDGE('',*,*,#35695,.T.);
#49674=ORIENTED_EDGE('',*,*,#35696,.F.);
#49675=ORIENTED_EDGE('',*,*,#35697,.T.);
#49676=ORIENTED_EDGE('',*,*,#35698,.T.);
#49677=ORIENTED_EDGE('',*,*,#35699,.F.);
#49678=ORIENTED_EDGE('',*,*,#35700,.T.);
#49679=ORIENTED_EDGE('',*,*,#35701,.T.);
#49680=ORIENTED_EDGE('',*,*,#35702,.F.);
#49681=ORIENTED_EDGE('',*,*,#35703,.T.);
#49682=ORIENTED_EDGE('',*,*,#35704,.T.);
#49683=ORIENTED_EDGE('',*,*,#35705,.F.);
#49684=ORIENTED_EDGE('',*,*,#35706,.T.);
#49685=ORIENTED_EDGE('',*,*,#35707,.T.);
#49686=ORIENTED_EDGE('',*,*,#35708,.F.);
#49687=ORIENTED_EDGE('',*,*,#35709,.T.);
#49688=ORIENTED_EDGE('',*,*,#35710,.T.);
#49689=ORIENTED_EDGE('',*,*,#35711,.T.);
#49690=ORIENTED_EDGE('',*,*,#35710,.F.);
#49691=ORIENTED_EDGE('',*,*,#35712,.T.);
#49692=ORIENTED_EDGE('',*,*,#35713,.F.);
#49693=ORIENTED_EDGE('',*,*,#35714,.T.);
#49694=ORIENTED_EDGE('',*,*,#35715,.T.);
#49695=ORIENTED_EDGE('',*,*,#35716,.F.);
#49696=ORIENTED_EDGE('',*,*,#35717,.T.);
#49697=ORIENTED_EDGE('',*,*,#35718,.T.);
#49698=ORIENTED_EDGE('',*,*,#35719,.F.);
#49699=ORIENTED_EDGE('',*,*,#35720,.T.);
#49700=ORIENTED_EDGE('',*,*,#35721,.T.);
#49701=ORIENTED_EDGE('',*,*,#35722,.F.);
#49702=ORIENTED_EDGE('',*,*,#35723,.T.);
#49703=ORIENTED_EDGE('',*,*,#35724,.T.);
#49704=ORIENTED_EDGE('',*,*,#35725,.F.);
#49705=ORIENTED_EDGE('',*,*,#35726,.T.);
#49706=ORIENTED_EDGE('',*,*,#35727,.T.);
#49707=ORIENTED_EDGE('',*,*,#35728,.F.);
#49708=ORIENTED_EDGE('',*,*,#35729,.T.);
#49709=ORIENTED_EDGE('',*,*,#35730,.T.);
#49710=ORIENTED_EDGE('',*,*,#35731,.F.);
#49711=ORIENTED_EDGE('',*,*,#35732,.T.);
#49712=ORIENTED_EDGE('',*,*,#35733,.T.);
#49713=ORIENTED_EDGE('',*,*,#35734,.F.);
#49714=ORIENTED_EDGE('',*,*,#35735,.T.);
#49715=ORIENTED_EDGE('',*,*,#35736,.T.);
#49716=ORIENTED_EDGE('',*,*,#35737,.F.);
#49717=ORIENTED_EDGE('',*,*,#35738,.T.);
#49718=ORIENTED_EDGE('',*,*,#35739,.T.);
#49719=ORIENTED_EDGE('',*,*,#35740,.F.);
#49720=ORIENTED_EDGE('',*,*,#35741,.T.);
#49721=ORIENTED_EDGE('',*,*,#35742,.T.);
#49722=ORIENTED_EDGE('',*,*,#35743,.F.);
#49723=ORIENTED_EDGE('',*,*,#35744,.T.);
#49724=ORIENTED_EDGE('',*,*,#35745,.T.);
#49725=ORIENTED_EDGE('',*,*,#35746,.F.);
#49726=ORIENTED_EDGE('',*,*,#35747,.T.);
#49727=ORIENTED_EDGE('',*,*,#35748,.T.);
#49728=ORIENTED_EDGE('',*,*,#35749,.F.);
#49729=ORIENTED_EDGE('',*,*,#35750,.T.);
#49730=ORIENTED_EDGE('',*,*,#35751,.T.);
#49731=ORIENTED_EDGE('',*,*,#35752,.F.);
#49732=ORIENTED_EDGE('',*,*,#35753,.T.);
#49733=ORIENTED_EDGE('',*,*,#35754,.T.);
#49734=ORIENTED_EDGE('',*,*,#35755,.F.);
#49735=ORIENTED_EDGE('',*,*,#35756,.T.);
#49736=ORIENTED_EDGE('',*,*,#35757,.T.);
#49737=ORIENTED_EDGE('',*,*,#35758,.F.);
#49738=ORIENTED_EDGE('',*,*,#35759,.T.);
#49739=ORIENTED_EDGE('',*,*,#35760,.T.);
#49740=ORIENTED_EDGE('',*,*,#35761,.F.);
#49741=ORIENTED_EDGE('',*,*,#35762,.T.);
#49742=ORIENTED_EDGE('',*,*,#35763,.T.);
#49743=ORIENTED_EDGE('',*,*,#35764,.F.);
#49744=ORIENTED_EDGE('',*,*,#35765,.T.);
#49745=ORIENTED_EDGE('',*,*,#35766,.T.);
#49746=ORIENTED_EDGE('',*,*,#35767,.F.);
#49747=ORIENTED_EDGE('',*,*,#35768,.T.);
#49748=ORIENTED_EDGE('',*,*,#35769,.T.);
#49749=ORIENTED_EDGE('',*,*,#35770,.F.);
#49750=ORIENTED_EDGE('',*,*,#35771,.T.);
#49751=ORIENTED_EDGE('',*,*,#35772,.T.);
#49752=ORIENTED_EDGE('',*,*,#35773,.F.);
#49753=ORIENTED_EDGE('',*,*,#35652,.T.);
#49754=ORIENTED_EDGE('',*,*,#35774,.F.);
#49755=ORIENTED_EDGE('',*,*,#35775,.T.);
#49756=ORIENTED_EDGE('',*,*,#35654,.T.);
#49757=ORIENTED_EDGE('',*,*,#35650,.T.);
#49758=ORIENTED_EDGE('',*,*,#35773,.T.);
#49759=ORIENTED_EDGE('',*,*,#35776,.T.);
#49760=ORIENTED_EDGE('',*,*,#35777,.F.);
#49761=ORIENTED_EDGE('',*,*,#35656,.F.);
#49762=ORIENTED_EDGE('',*,*,#35778,.F.);
#49763=ORIENTED_EDGE('',*,*,#35779,.F.);
#49764=ORIENTED_EDGE('',*,*,#35780,.F.);
#49765=ORIENTED_EDGE('',*,*,#35655,.F.);
#49766=ORIENTED_EDGE('',*,*,#35775,.F.);
#49767=ORIENTED_EDGE('',*,*,#35781,.F.);
#49768=ORIENTED_EDGE('',*,*,#35778,.T.);
#49769=ORIENTED_EDGE('',*,*,#35780,.T.);
#49770=ORIENTED_EDGE('',*,*,#35782,.F.);
#49771=ORIENTED_EDGE('',*,*,#35783,.T.);
#49772=ORIENTED_EDGE('',*,*,#35657,.T.);
#49773=ORIENTED_EDGE('',*,*,#35784,.F.);
#49774=ORIENTED_EDGE('',*,*,#35785,.T.);
#49775=ORIENTED_EDGE('',*,*,#35786,.T.);
#49776=ORIENTED_EDGE('',*,*,#35787,.T.);
#49777=ORIENTED_EDGE('',*,*,#35788,.T.);
#49778=ORIENTED_EDGE('',*,*,#35789,.T.);
#49779=ORIENTED_EDGE('',*,*,#35790,.T.);
#49780=ORIENTED_EDGE('',*,*,#35791,.T.);
#49781=ORIENTED_EDGE('',*,*,#35792,.T.);
#49782=ORIENTED_EDGE('',*,*,#35793,.T.);
#49783=ORIENTED_EDGE('',*,*,#35794,.T.);
#49784=ORIENTED_EDGE('',*,*,#35795,.T.);
#49785=ORIENTED_EDGE('',*,*,#35796,.T.);
#49786=ORIENTED_EDGE('',*,*,#35797,.T.);
#49787=ORIENTED_EDGE('',*,*,#35798,.T.);
#49788=ORIENTED_EDGE('',*,*,#35799,.T.);
#49789=ORIENTED_EDGE('',*,*,#35800,.T.);
#49790=ORIENTED_EDGE('',*,*,#35801,.T.);
#49791=ORIENTED_EDGE('',*,*,#35802,.T.);
#49792=ORIENTED_EDGE('',*,*,#35803,.T.);
#49793=ORIENTED_EDGE('',*,*,#35804,.T.);
#49794=ORIENTED_EDGE('',*,*,#35805,.T.);
#49795=ORIENTED_EDGE('',*,*,#35806,.T.);
#49796=ORIENTED_EDGE('',*,*,#35807,.T.);
#49797=ORIENTED_EDGE('',*,*,#35808,.T.);
#49798=ORIENTED_EDGE('',*,*,#35809,.T.);
#49799=ORIENTED_EDGE('',*,*,#35810,.T.);
#49800=ORIENTED_EDGE('',*,*,#35811,.T.);
#49801=ORIENTED_EDGE('',*,*,#35812,.T.);
#49802=ORIENTED_EDGE('',*,*,#35813,.T.);
#49803=ORIENTED_EDGE('',*,*,#35814,.T.);
#49804=ORIENTED_EDGE('',*,*,#35815,.T.);
#49805=ORIENTED_EDGE('',*,*,#35816,.T.);
#49806=ORIENTED_EDGE('',*,*,#35817,.T.);
#49807=ORIENTED_EDGE('',*,*,#35818,.T.);
#49808=ORIENTED_EDGE('',*,*,#35819,.T.);
#49809=ORIENTED_EDGE('',*,*,#35820,.T.);
#49810=ORIENTED_EDGE('',*,*,#35821,.T.);
#49811=ORIENTED_EDGE('',*,*,#35822,.T.);
#49812=ORIENTED_EDGE('',*,*,#35823,.T.);
#49813=ORIENTED_EDGE('',*,*,#35824,.T.);
#49814=ORIENTED_EDGE('',*,*,#35825,.T.);
#49815=ORIENTED_EDGE('',*,*,#35826,.T.);
#49816=ORIENTED_EDGE('',*,*,#35827,.T.);
#49817=ORIENTED_EDGE('',*,*,#35828,.T.);
#49818=ORIENTED_EDGE('',*,*,#35829,.T.);
#49819=ORIENTED_EDGE('',*,*,#35830,.T.);
#49820=ORIENTED_EDGE('',*,*,#35831,.T.);
#49821=ORIENTED_EDGE('',*,*,#35832,.T.);
#49822=ORIENTED_EDGE('',*,*,#35833,.T.);
#49823=ORIENTED_EDGE('',*,*,#35834,.T.);
#49824=ORIENTED_EDGE('',*,*,#35835,.T.);
#49825=ORIENTED_EDGE('',*,*,#35836,.T.);
#49826=ORIENTED_EDGE('',*,*,#35837,.T.);
#49827=ORIENTED_EDGE('',*,*,#35782,.T.);
#49828=ORIENTED_EDGE('',*,*,#35779,.T.);
#49829=ORIENTED_EDGE('',*,*,#35781,.T.);
#49830=ORIENTED_EDGE('',*,*,#35774,.T.);
#49831=ORIENTED_EDGE('',*,*,#35651,.T.);
#49832=ORIENTED_EDGE('',*,*,#35647,.T.);
#49833=ORIENTED_EDGE('',*,*,#35777,.T.);
#49834=ORIENTED_EDGE('',*,*,#35838,.T.);
#49835=ORIENTED_EDGE('',*,*,#35839,.T.);
#49836=ORIENTED_EDGE('',*,*,#35840,.T.);
#49837=ORIENTED_EDGE('',*,*,#35841,.T.);
#49838=ORIENTED_EDGE('',*,*,#35842,.T.);
#49839=ORIENTED_EDGE('',*,*,#35843,.T.);
#49840=ORIENTED_EDGE('',*,*,#35844,.T.);
#49841=ORIENTED_EDGE('',*,*,#35845,.T.);
#49842=ORIENTED_EDGE('',*,*,#35846,.T.);
#49843=ORIENTED_EDGE('',*,*,#35847,.T.);
#49844=ORIENTED_EDGE('',*,*,#35848,.T.);
#49845=ORIENTED_EDGE('',*,*,#35849,.T.);
#49846=ORIENTED_EDGE('',*,*,#35850,.T.);
#49847=ORIENTED_EDGE('',*,*,#35851,.T.);
#49848=ORIENTED_EDGE('',*,*,#35852,.T.);
#49849=ORIENTED_EDGE('',*,*,#35853,.T.);
#49850=ORIENTED_EDGE('',*,*,#35854,.T.);
#49851=ORIENTED_EDGE('',*,*,#35855,.T.);
#49852=ORIENTED_EDGE('',*,*,#35856,.T.);
#49853=ORIENTED_EDGE('',*,*,#35857,.T.);
#49854=ORIENTED_EDGE('',*,*,#35858,.T.);
#49855=ORIENTED_EDGE('',*,*,#35859,.T.);
#49856=ORIENTED_EDGE('',*,*,#35860,.T.);
#49857=ORIENTED_EDGE('',*,*,#35861,.T.);
#49858=ORIENTED_EDGE('',*,*,#35862,.T.);
#49859=ORIENTED_EDGE('',*,*,#35863,.T.);
#49860=ORIENTED_EDGE('',*,*,#35864,.T.);
#49861=ORIENTED_EDGE('',*,*,#35865,.T.);
#49862=ORIENTED_EDGE('',*,*,#35866,.T.);
#49863=ORIENTED_EDGE('',*,*,#35867,.T.);
#49864=ORIENTED_EDGE('',*,*,#35868,.T.);
#49865=ORIENTED_EDGE('',*,*,#35869,.T.);
#49866=ORIENTED_EDGE('',*,*,#35870,.T.);
#49867=ORIENTED_EDGE('',*,*,#35871,.T.);
#49868=ORIENTED_EDGE('',*,*,#35872,.T.);
#49869=ORIENTED_EDGE('',*,*,#35873,.T.);
#49870=ORIENTED_EDGE('',*,*,#35874,.T.);
#49871=ORIENTED_EDGE('',*,*,#35875,.T.);
#49872=ORIENTED_EDGE('',*,*,#35876,.T.);
#49873=ORIENTED_EDGE('',*,*,#35877,.T.);
#49874=ORIENTED_EDGE('',*,*,#35878,.T.);
#49875=ORIENTED_EDGE('',*,*,#35879,.T.);
#49876=ORIENTED_EDGE('',*,*,#35880,.T.);
#49877=ORIENTED_EDGE('',*,*,#35881,.T.);
#49878=ORIENTED_EDGE('',*,*,#35882,.T.);
#49879=ORIENTED_EDGE('',*,*,#35883,.T.);
#49880=ORIENTED_EDGE('',*,*,#35884,.T.);
#49881=ORIENTED_EDGE('',*,*,#35885,.T.);
#49882=ORIENTED_EDGE('',*,*,#35886,.T.);
#49883=ORIENTED_EDGE('',*,*,#35887,.T.);
#49884=ORIENTED_EDGE('',*,*,#35888,.T.);
#49885=ORIENTED_EDGE('',*,*,#35889,.T.);
#49886=ORIENTED_EDGE('',*,*,#35890,.T.);
#49887=ORIENTED_EDGE('',*,*,#35891,.T.);
#49888=ORIENTED_EDGE('',*,*,#35892,.T.);
#49889=ORIENTED_EDGE('',*,*,#35893,.T.);
#49890=ORIENTED_EDGE('',*,*,#35894,.T.);
#49891=ORIENTED_EDGE('',*,*,#35895,.T.);
#49892=ORIENTED_EDGE('',*,*,#35896,.T.);
#49893=ORIENTED_EDGE('',*,*,#35897,.T.);
#49894=ORIENTED_EDGE('',*,*,#35898,.T.);
#49895=ORIENTED_EDGE('',*,*,#35785,.F.);
#49896=ORIENTED_EDGE('',*,*,#35837,.F.);
#49897=ORIENTED_EDGE('',*,*,#35899,.T.);
#49898=ORIENTED_EDGE('',*,*,#35658,.F.);
#49899=ORIENTED_EDGE('',*,*,#35783,.F.);
#49900=ORIENTED_EDGE('',*,*,#35836,.F.);
#49901=ORIENTED_EDGE('',*,*,#35900,.F.);
#49902=ORIENTED_EDGE('',*,*,#35659,.F.);
#49903=ORIENTED_EDGE('',*,*,#35899,.F.);
#49904=ORIENTED_EDGE('',*,*,#35834,.F.);
#49905=ORIENTED_EDGE('',*,*,#35901,.T.);
#49906=ORIENTED_EDGE('',*,*,#35661,.F.);
#49907=ORIENTED_EDGE('',*,*,#35902,.F.);
#49908=ORIENTED_EDGE('',*,*,#35833,.F.);
#49909=ORIENTED_EDGE('',*,*,#35903,.F.);
#49910=ORIENTED_EDGE('',*,*,#35662,.F.);
#49911=ORIENTED_EDGE('',*,*,#35901,.F.);
#49912=ORIENTED_EDGE('',*,*,#35903,.T.);
#49913=ORIENTED_EDGE('',*,*,#35832,.F.);
#49914=ORIENTED_EDGE('',*,*,#35904,.T.);
#49915=ORIENTED_EDGE('',*,*,#35663,.T.);
#49916=ORIENTED_EDGE('',*,*,#35900,.T.);
#49917=ORIENTED_EDGE('',*,*,#35835,.F.);
#49918=ORIENTED_EDGE('',*,*,#35902,.T.);
#49919=ORIENTED_EDGE('',*,*,#35660,.T.);
#49920=ORIENTED_EDGE('',*,*,#35665,.F.);
#49921=ORIENTED_EDGE('',*,*,#35905,.F.);
#49922=ORIENTED_EDGE('',*,*,#35830,.F.);
#49923=ORIENTED_EDGE('',*,*,#35906,.F.);
#49924=ORIENTED_EDGE('',*,*,#35664,.F.);
#49925=ORIENTED_EDGE('',*,*,#35904,.F.);
#49926=ORIENTED_EDGE('',*,*,#35831,.F.);
#49927=ORIENTED_EDGE('',*,*,#35905,.T.);
#49928=ORIENTED_EDGE('',*,*,#35906,.T.);
#49929=ORIENTED_EDGE('',*,*,#35829,.F.);
#49930=ORIENTED_EDGE('',*,*,#35907,.T.);
#49931=ORIENTED_EDGE('',*,*,#35666,.T.);
#49932=ORIENTED_EDGE('',*,*,#35828,.F.);
#49933=ORIENTED_EDGE('',*,*,#35908,.T.);
#49934=ORIENTED_EDGE('',*,*,#35667,.F.);
#49935=ORIENTED_EDGE('',*,*,#35907,.F.);
#49936=ORIENTED_EDGE('',*,*,#35827,.F.);
#49937=ORIENTED_EDGE('',*,*,#35909,.F.);
#49938=ORIENTED_EDGE('',*,*,#35668,.F.);
#49939=ORIENTED_EDGE('',*,*,#35908,.F.);
#49940=ORIENTED_EDGE('',*,*,#35825,.F.);
#49941=ORIENTED_EDGE('',*,*,#35910,.T.);
#49942=ORIENTED_EDGE('',*,*,#35670,.F.);
#49943=ORIENTED_EDGE('',*,*,#35911,.F.);
#49944=ORIENTED_EDGE('',*,*,#35824,.F.);
#49945=ORIENTED_EDGE('',*,*,#35912,.F.);
#49946=ORIENTED_EDGE('',*,*,#35671,.F.);
#49947=ORIENTED_EDGE('',*,*,#35910,.F.);
#49948=ORIENTED_EDGE('',*,*,#35912,.T.);
#49949=ORIENTED_EDGE('',*,*,#35823,.F.);
#49950=ORIENTED_EDGE('',*,*,#35913,.T.);
#49951=ORIENTED_EDGE('',*,*,#35672,.T.);
#49952=ORIENTED_EDGE('',*,*,#35909,.T.);
#49953=ORIENTED_EDGE('',*,*,#35826,.F.);
#49954=ORIENTED_EDGE('',*,*,#35911,.T.);
#49955=ORIENTED_EDGE('',*,*,#35669,.T.);
#49956=ORIENTED_EDGE('',*,*,#35674,.F.);
#49957=ORIENTED_EDGE('',*,*,#35914,.F.);
#49958=ORIENTED_EDGE('',*,*,#35821,.F.);
#49959=ORIENTED_EDGE('',*,*,#35915,.F.);
#49960=ORIENTED_EDGE('',*,*,#35673,.F.);
#49961=ORIENTED_EDGE('',*,*,#35913,.F.);
#49962=ORIENTED_EDGE('',*,*,#35822,.F.);
#49963=ORIENTED_EDGE('',*,*,#35914,.T.);
#49964=ORIENTED_EDGE('',*,*,#35915,.T.);
#49965=ORIENTED_EDGE('',*,*,#35820,.F.);
#49966=ORIENTED_EDGE('',*,*,#35916,.T.);
#49967=ORIENTED_EDGE('',*,*,#35675,.T.);
#49968=ORIENTED_EDGE('',*,*,#35819,.F.);
#49969=ORIENTED_EDGE('',*,*,#35917,.T.);
#49970=ORIENTED_EDGE('',*,*,#35676,.F.);
#49971=ORIENTED_EDGE('',*,*,#35916,.F.);
#49972=ORIENTED_EDGE('',*,*,#35818,.F.);
#49973=ORIENTED_EDGE('',*,*,#35918,.F.);
#49974=ORIENTED_EDGE('',*,*,#35677,.F.);
#49975=ORIENTED_EDGE('',*,*,#35917,.F.);
#49976=ORIENTED_EDGE('',*,*,#35816,.F.);
#49977=ORIENTED_EDGE('',*,*,#35919,.T.);
#49978=ORIENTED_EDGE('',*,*,#35679,.F.);
#49979=ORIENTED_EDGE('',*,*,#35920,.F.);
#49980=ORIENTED_EDGE('',*,*,#35815,.F.);
#49981=ORIENTED_EDGE('',*,*,#35921,.F.);
#49982=ORIENTED_EDGE('',*,*,#35680,.F.);
#49983=ORIENTED_EDGE('',*,*,#35919,.F.);
#49984=ORIENTED_EDGE('',*,*,#35921,.T.);
#49985=ORIENTED_EDGE('',*,*,#35814,.F.);
#49986=ORIENTED_EDGE('',*,*,#35922,.T.);
#49987=ORIENTED_EDGE('',*,*,#35681,.T.);
#49988=ORIENTED_EDGE('',*,*,#35918,.T.);
#49989=ORIENTED_EDGE('',*,*,#35817,.F.);
#49990=ORIENTED_EDGE('',*,*,#35920,.T.);
#49991=ORIENTED_EDGE('',*,*,#35678,.T.);
#49992=ORIENTED_EDGE('',*,*,#35683,.F.);
#49993=ORIENTED_EDGE('',*,*,#35923,.F.);
#49994=ORIENTED_EDGE('',*,*,#35812,.F.);
#49995=ORIENTED_EDGE('',*,*,#35924,.F.);
#49996=ORIENTED_EDGE('',*,*,#35682,.F.);
#49997=ORIENTED_EDGE('',*,*,#35922,.F.);
#49998=ORIENTED_EDGE('',*,*,#35813,.F.);
#49999=ORIENTED_EDGE('',*,*,#35923,.T.);
#50000=ORIENTED_EDGE('',*,*,#35924,.T.);
#50001=ORIENTED_EDGE('',*,*,#35811,.F.);
#50002=ORIENTED_EDGE('',*,*,#35925,.T.);
#50003=ORIENTED_EDGE('',*,*,#35684,.T.);
#50004=ORIENTED_EDGE('',*,*,#35810,.F.);
#50005=ORIENTED_EDGE('',*,*,#35926,.T.);
#50006=ORIENTED_EDGE('',*,*,#35685,.F.);
#50007=ORIENTED_EDGE('',*,*,#35925,.F.);
#50008=ORIENTED_EDGE('',*,*,#35809,.F.);
#50009=ORIENTED_EDGE('',*,*,#35927,.F.);
#50010=ORIENTED_EDGE('',*,*,#35686,.F.);
#50011=ORIENTED_EDGE('',*,*,#35926,.F.);
#50012=ORIENTED_EDGE('',*,*,#35807,.F.);
#50013=ORIENTED_EDGE('',*,*,#35928,.T.);
#50014=ORIENTED_EDGE('',*,*,#35688,.F.);
#50015=ORIENTED_EDGE('',*,*,#35929,.F.);
#50016=ORIENTED_EDGE('',*,*,#35806,.F.);
#50017=ORIENTED_EDGE('',*,*,#35930,.F.);
#50018=ORIENTED_EDGE('',*,*,#35689,.F.);
#50019=ORIENTED_EDGE('',*,*,#35928,.F.);
#50020=ORIENTED_EDGE('',*,*,#35930,.T.);
#50021=ORIENTED_EDGE('',*,*,#35805,.F.);
#50022=ORIENTED_EDGE('',*,*,#35931,.T.);
#50023=ORIENTED_EDGE('',*,*,#35690,.T.);
#50024=ORIENTED_EDGE('',*,*,#35927,.T.);
#50025=ORIENTED_EDGE('',*,*,#35808,.F.);
#50026=ORIENTED_EDGE('',*,*,#35929,.T.);
#50027=ORIENTED_EDGE('',*,*,#35687,.T.);
#50028=ORIENTED_EDGE('',*,*,#35692,.F.);
#50029=ORIENTED_EDGE('',*,*,#35932,.F.);
#50030=ORIENTED_EDGE('',*,*,#35803,.F.);
#50031=ORIENTED_EDGE('',*,*,#35933,.F.);
#50032=ORIENTED_EDGE('',*,*,#35691,.F.);
#50033=ORIENTED_EDGE('',*,*,#35931,.F.);
#50034=ORIENTED_EDGE('',*,*,#35804,.F.);
#50035=ORIENTED_EDGE('',*,*,#35932,.T.);
#50036=ORIENTED_EDGE('',*,*,#35933,.T.);
#50037=ORIENTED_EDGE('',*,*,#35802,.F.);
#50038=ORIENTED_EDGE('',*,*,#35934,.T.);
#50039=ORIENTED_EDGE('',*,*,#35693,.T.);
#50040=ORIENTED_EDGE('',*,*,#35801,.F.);
#50041=ORIENTED_EDGE('',*,*,#35935,.T.);
#50042=ORIENTED_EDGE('',*,*,#35694,.F.);
#50043=ORIENTED_EDGE('',*,*,#35934,.F.);
#50044=ORIENTED_EDGE('',*,*,#35800,.F.);
#50045=ORIENTED_EDGE('',*,*,#35936,.F.);
#50046=ORIENTED_EDGE('',*,*,#35695,.F.);
#50047=ORIENTED_EDGE('',*,*,#35935,.F.);
#50048=ORIENTED_EDGE('',*,*,#35798,.F.);
#50049=ORIENTED_EDGE('',*,*,#35937,.T.);
#50050=ORIENTED_EDGE('',*,*,#35697,.F.);
#50051=ORIENTED_EDGE('',*,*,#35938,.F.);
#50052=ORIENTED_EDGE('',*,*,#35797,.F.);
#50053=ORIENTED_EDGE('',*,*,#35939,.F.);
#50054=ORIENTED_EDGE('',*,*,#35698,.F.);
#50055=ORIENTED_EDGE('',*,*,#35937,.F.);
#50056=ORIENTED_EDGE('',*,*,#35939,.T.);
#50057=ORIENTED_EDGE('',*,*,#35796,.F.);
#50058=ORIENTED_EDGE('',*,*,#35940,.T.);
#50059=ORIENTED_EDGE('',*,*,#35699,.T.);
#50060=ORIENTED_EDGE('',*,*,#35936,.T.);
#50061=ORIENTED_EDGE('',*,*,#35799,.F.);
#50062=ORIENTED_EDGE('',*,*,#35938,.T.);
#50063=ORIENTED_EDGE('',*,*,#35696,.T.);
#50064=ORIENTED_EDGE('',*,*,#35701,.F.);
#50065=ORIENTED_EDGE('',*,*,#35941,.F.);
#50066=ORIENTED_EDGE('',*,*,#35794,.F.);
#50067=ORIENTED_EDGE('',*,*,#35942,.F.);
#50068=ORIENTED_EDGE('',*,*,#35700,.F.);
#50069=ORIENTED_EDGE('',*,*,#35940,.F.);
#50070=ORIENTED_EDGE('',*,*,#35795,.F.);
#50071=ORIENTED_EDGE('',*,*,#35941,.T.);
#50072=ORIENTED_EDGE('',*,*,#35942,.T.);
#50073=ORIENTED_EDGE('',*,*,#35793,.F.);
#50074=ORIENTED_EDGE('',*,*,#35943,.T.);
#50075=ORIENTED_EDGE('',*,*,#35702,.T.);
#50076=ORIENTED_EDGE('',*,*,#35792,.F.);
#50077=ORIENTED_EDGE('',*,*,#35944,.T.);
#50078=ORIENTED_EDGE('',*,*,#35703,.F.);
#50079=ORIENTED_EDGE('',*,*,#35943,.F.);
#50080=ORIENTED_EDGE('',*,*,#35791,.F.);
#50081=ORIENTED_EDGE('',*,*,#35945,.F.);
#50082=ORIENTED_EDGE('',*,*,#35704,.F.);
#50083=ORIENTED_EDGE('',*,*,#35944,.F.);
#50084=ORIENTED_EDGE('',*,*,#35789,.F.);
#50085=ORIENTED_EDGE('',*,*,#35946,.T.);
#50086=ORIENTED_EDGE('',*,*,#35706,.F.);
#50087=ORIENTED_EDGE('',*,*,#35947,.F.);
#50088=ORIENTED_EDGE('',*,*,#35788,.F.);
#50089=ORIENTED_EDGE('',*,*,#35948,.F.);
#50090=ORIENTED_EDGE('',*,*,#35707,.F.);
#50091=ORIENTED_EDGE('',*,*,#35946,.F.);
#50092=ORIENTED_EDGE('',*,*,#35948,.T.);
#50093=ORIENTED_EDGE('',*,*,#35787,.F.);
#50094=ORIENTED_EDGE('',*,*,#35949,.T.);
#50095=ORIENTED_EDGE('',*,*,#35708,.T.);
#50096=ORIENTED_EDGE('',*,*,#35945,.T.);
#50097=ORIENTED_EDGE('',*,*,#35790,.F.);
#50098=ORIENTED_EDGE('',*,*,#35947,.T.);
#50099=ORIENTED_EDGE('',*,*,#35705,.T.);
#50100=ORIENTED_EDGE('',*,*,#35712,.F.);
#50101=ORIENTED_EDGE('',*,*,#35950,.F.);
#50102=ORIENTED_EDGE('',*,*,#35898,.F.);
#50103=ORIENTED_EDGE('',*,*,#35951,.F.);
#50104=ORIENTED_EDGE('',*,*,#35709,.F.);
#50105=ORIENTED_EDGE('',*,*,#35949,.F.);
#50106=ORIENTED_EDGE('',*,*,#35786,.F.);
#50107=ORIENTED_EDGE('',*,*,#35950,.T.);
#50108=ORIENTED_EDGE('',*,*,#35951,.T.);
#50109=ORIENTED_EDGE('',*,*,#35897,.F.);
#50110=ORIENTED_EDGE('',*,*,#35952,.T.);
#50111=ORIENTED_EDGE('',*,*,#35713,.T.);
#50112=ORIENTED_EDGE('',*,*,#35896,.F.);
#50113=ORIENTED_EDGE('',*,*,#35953,.T.);
#50114=ORIENTED_EDGE('',*,*,#35714,.F.);
#50115=ORIENTED_EDGE('',*,*,#35952,.F.);
#50116=ORIENTED_EDGE('',*,*,#35895,.F.);
#50117=ORIENTED_EDGE('',*,*,#35954,.F.);
#50118=ORIENTED_EDGE('',*,*,#35715,.F.);
#50119=ORIENTED_EDGE('',*,*,#35953,.F.);
#50120=ORIENTED_EDGE('',*,*,#35893,.F.);
#50121=ORIENTED_EDGE('',*,*,#35955,.T.);
#50122=ORIENTED_EDGE('',*,*,#35717,.F.);
#50123=ORIENTED_EDGE('',*,*,#35956,.F.);
#50124=ORIENTED_EDGE('',*,*,#35892,.F.);
#50125=ORIENTED_EDGE('',*,*,#35957,.F.);
#50126=ORIENTED_EDGE('',*,*,#35718,.F.);
#50127=ORIENTED_EDGE('',*,*,#35955,.F.);
#50128=ORIENTED_EDGE('',*,*,#35957,.T.);
#50129=ORIENTED_EDGE('',*,*,#35891,.F.);
#50130=ORIENTED_EDGE('',*,*,#35958,.T.);
#50131=ORIENTED_EDGE('',*,*,#35719,.T.);
#50132=ORIENTED_EDGE('',*,*,#35954,.T.);
#50133=ORIENTED_EDGE('',*,*,#35894,.F.);
#50134=ORIENTED_EDGE('',*,*,#35956,.T.);
#50135=ORIENTED_EDGE('',*,*,#35716,.T.);
#50136=ORIENTED_EDGE('',*,*,#35721,.F.);
#50137=ORIENTED_EDGE('',*,*,#35959,.F.);
#50138=ORIENTED_EDGE('',*,*,#35889,.F.);
#50139=ORIENTED_EDGE('',*,*,#35960,.F.);
#50140=ORIENTED_EDGE('',*,*,#35720,.F.);
#50141=ORIENTED_EDGE('',*,*,#35958,.F.);
#50142=ORIENTED_EDGE('',*,*,#35890,.F.);
#50143=ORIENTED_EDGE('',*,*,#35959,.T.);
#50144=ORIENTED_EDGE('',*,*,#35960,.T.);
#50145=ORIENTED_EDGE('',*,*,#35888,.F.);
#50146=ORIENTED_EDGE('',*,*,#35961,.T.);
#50147=ORIENTED_EDGE('',*,*,#35722,.T.);
#50148=ORIENTED_EDGE('',*,*,#35887,.F.);
#50149=ORIENTED_EDGE('',*,*,#35962,.T.);
#50150=ORIENTED_EDGE('',*,*,#35723,.F.);
#50151=ORIENTED_EDGE('',*,*,#35961,.F.);
#50152=ORIENTED_EDGE('',*,*,#35886,.F.);
#50153=ORIENTED_EDGE('',*,*,#35963,.F.);
#50154=ORIENTED_EDGE('',*,*,#35724,.F.);
#50155=ORIENTED_EDGE('',*,*,#35962,.F.);
#50156=ORIENTED_EDGE('',*,*,#35884,.F.);
#50157=ORIENTED_EDGE('',*,*,#35964,.T.);
#50158=ORIENTED_EDGE('',*,*,#35726,.F.);
#50159=ORIENTED_EDGE('',*,*,#35965,.F.);
#50160=ORIENTED_EDGE('',*,*,#35883,.F.);
#50161=ORIENTED_EDGE('',*,*,#35966,.F.);
#50162=ORIENTED_EDGE('',*,*,#35727,.F.);
#50163=ORIENTED_EDGE('',*,*,#35964,.F.);
#50164=ORIENTED_EDGE('',*,*,#35966,.T.);
#50165=ORIENTED_EDGE('',*,*,#35882,.F.);
#50166=ORIENTED_EDGE('',*,*,#35967,.T.);
#50167=ORIENTED_EDGE('',*,*,#35728,.T.);
#50168=ORIENTED_EDGE('',*,*,#35963,.T.);
#50169=ORIENTED_EDGE('',*,*,#35885,.F.);
#50170=ORIENTED_EDGE('',*,*,#35965,.T.);
#50171=ORIENTED_EDGE('',*,*,#35725,.T.);
#50172=ORIENTED_EDGE('',*,*,#35730,.F.);
#50173=ORIENTED_EDGE('',*,*,#35968,.F.);
#50174=ORIENTED_EDGE('',*,*,#35880,.F.);
#50175=ORIENTED_EDGE('',*,*,#35969,.F.);
#50176=ORIENTED_EDGE('',*,*,#35729,.F.);
#50177=ORIENTED_EDGE('',*,*,#35967,.F.);
#50178=ORIENTED_EDGE('',*,*,#35881,.F.);
#50179=ORIENTED_EDGE('',*,*,#35968,.T.);
#50180=ORIENTED_EDGE('',*,*,#35969,.T.);
#50181=ORIENTED_EDGE('',*,*,#35879,.F.);
#50182=ORIENTED_EDGE('',*,*,#35970,.T.);
#50183=ORIENTED_EDGE('',*,*,#35731,.T.);
#50184=ORIENTED_EDGE('',*,*,#35878,.F.);
#50185=ORIENTED_EDGE('',*,*,#35971,.T.);
#50186=ORIENTED_EDGE('',*,*,#35732,.F.);
#50187=ORIENTED_EDGE('',*,*,#35970,.F.);
#50188=ORIENTED_EDGE('',*,*,#35877,.F.);
#50189=ORIENTED_EDGE('',*,*,#35972,.F.);
#50190=ORIENTED_EDGE('',*,*,#35733,.F.);
#50191=ORIENTED_EDGE('',*,*,#35971,.F.);
#50192=ORIENTED_EDGE('',*,*,#35875,.F.);
#50193=ORIENTED_EDGE('',*,*,#35973,.T.);
#50194=ORIENTED_EDGE('',*,*,#35735,.F.);
#50195=ORIENTED_EDGE('',*,*,#35974,.F.);
#50196=ORIENTED_EDGE('',*,*,#35874,.F.);
#50197=ORIENTED_EDGE('',*,*,#35975,.F.);
#50198=ORIENTED_EDGE('',*,*,#35736,.F.);
#50199=ORIENTED_EDGE('',*,*,#35973,.F.);
#50200=ORIENTED_EDGE('',*,*,#35975,.T.);
#50201=ORIENTED_EDGE('',*,*,#35873,.F.);
#50202=ORIENTED_EDGE('',*,*,#35976,.T.);
#50203=ORIENTED_EDGE('',*,*,#35737,.T.);
#50204=ORIENTED_EDGE('',*,*,#35972,.T.);
#50205=ORIENTED_EDGE('',*,*,#35876,.F.);
#50206=ORIENTED_EDGE('',*,*,#35974,.T.);
#50207=ORIENTED_EDGE('',*,*,#35734,.T.);
#50208=ORIENTED_EDGE('',*,*,#35739,.F.);
#50209=ORIENTED_EDGE('',*,*,#35977,.F.);
#50210=ORIENTED_EDGE('',*,*,#35871,.F.);
#50211=ORIENTED_EDGE('',*,*,#35978,.F.);
#50212=ORIENTED_EDGE('',*,*,#35738,.F.);
#50213=ORIENTED_EDGE('',*,*,#35976,.F.);
#50214=ORIENTED_EDGE('',*,*,#35872,.F.);
#50215=ORIENTED_EDGE('',*,*,#35977,.T.);
#50216=ORIENTED_EDGE('',*,*,#35978,.T.);
#50217=ORIENTED_EDGE('',*,*,#35870,.F.);
#50218=ORIENTED_EDGE('',*,*,#35979,.T.);
#50219=ORIENTED_EDGE('',*,*,#35740,.T.);
#50220=ORIENTED_EDGE('',*,*,#35869,.F.);
#50221=ORIENTED_EDGE('',*,*,#35980,.T.);
#50222=ORIENTED_EDGE('',*,*,#35741,.F.);
#50223=ORIENTED_EDGE('',*,*,#35979,.F.);
#50224=ORIENTED_EDGE('',*,*,#35868,.F.);
#50225=ORIENTED_EDGE('',*,*,#35981,.F.);
#50226=ORIENTED_EDGE('',*,*,#35742,.F.);
#50227=ORIENTED_EDGE('',*,*,#35980,.F.);
#50228=ORIENTED_EDGE('',*,*,#35866,.F.);
#50229=ORIENTED_EDGE('',*,*,#35982,.T.);
#50230=ORIENTED_EDGE('',*,*,#35744,.F.);
#50231=ORIENTED_EDGE('',*,*,#35983,.F.);
#50232=ORIENTED_EDGE('',*,*,#35865,.F.);
#50233=ORIENTED_EDGE('',*,*,#35984,.F.);
#50234=ORIENTED_EDGE('',*,*,#35745,.F.);
#50235=ORIENTED_EDGE('',*,*,#35982,.F.);
#50236=ORIENTED_EDGE('',*,*,#35984,.T.);
#50237=ORIENTED_EDGE('',*,*,#35864,.F.);
#50238=ORIENTED_EDGE('',*,*,#35985,.T.);
#50239=ORIENTED_EDGE('',*,*,#35746,.T.);
#50240=ORIENTED_EDGE('',*,*,#35981,.T.);
#50241=ORIENTED_EDGE('',*,*,#35867,.F.);
#50242=ORIENTED_EDGE('',*,*,#35983,.T.);
#50243=ORIENTED_EDGE('',*,*,#35743,.T.);
#50244=ORIENTED_EDGE('',*,*,#35748,.F.);
#50245=ORIENTED_EDGE('',*,*,#35986,.F.);
#50246=ORIENTED_EDGE('',*,*,#35862,.F.);
#50247=ORIENTED_EDGE('',*,*,#35987,.F.);
#50248=ORIENTED_EDGE('',*,*,#35747,.F.);
#50249=ORIENTED_EDGE('',*,*,#35985,.F.);
#50250=ORIENTED_EDGE('',*,*,#35863,.F.);
#50251=ORIENTED_EDGE('',*,*,#35986,.T.);
#50252=ORIENTED_EDGE('',*,*,#35987,.T.);
#50253=ORIENTED_EDGE('',*,*,#35861,.F.);
#50254=ORIENTED_EDGE('',*,*,#35988,.T.);
#50255=ORIENTED_EDGE('',*,*,#35749,.T.);
#50256=ORIENTED_EDGE('',*,*,#35860,.F.);
#50257=ORIENTED_EDGE('',*,*,#35989,.T.);
#50258=ORIENTED_EDGE('',*,*,#35750,.F.);
#50259=ORIENTED_EDGE('',*,*,#35988,.F.);
#50260=ORIENTED_EDGE('',*,*,#35859,.F.);
#50261=ORIENTED_EDGE('',*,*,#35990,.F.);
#50262=ORIENTED_EDGE('',*,*,#35751,.F.);
#50263=ORIENTED_EDGE('',*,*,#35989,.F.);
#50264=ORIENTED_EDGE('',*,*,#35857,.F.);
#50265=ORIENTED_EDGE('',*,*,#35991,.T.);
#50266=ORIENTED_EDGE('',*,*,#35753,.F.);
#50267=ORIENTED_EDGE('',*,*,#35992,.F.);
#50268=ORIENTED_EDGE('',*,*,#35856,.F.);
#50269=ORIENTED_EDGE('',*,*,#35993,.F.);
#50270=ORIENTED_EDGE('',*,*,#35754,.F.);
#50271=ORIENTED_EDGE('',*,*,#35991,.F.);
#50272=ORIENTED_EDGE('',*,*,#35993,.T.);
#50273=ORIENTED_EDGE('',*,*,#35855,.F.);
#50274=ORIENTED_EDGE('',*,*,#35994,.T.);
#50275=ORIENTED_EDGE('',*,*,#35755,.T.);
#50276=ORIENTED_EDGE('',*,*,#35990,.T.);
#50277=ORIENTED_EDGE('',*,*,#35858,.F.);
#50278=ORIENTED_EDGE('',*,*,#35992,.T.);
#50279=ORIENTED_EDGE('',*,*,#35752,.T.);
#50280=ORIENTED_EDGE('',*,*,#35757,.F.);
#50281=ORIENTED_EDGE('',*,*,#35995,.F.);
#50282=ORIENTED_EDGE('',*,*,#35853,.F.);
#50283=ORIENTED_EDGE('',*,*,#35996,.F.);
#50284=ORIENTED_EDGE('',*,*,#35756,.F.);
#50285=ORIENTED_EDGE('',*,*,#35994,.F.);
#50286=ORIENTED_EDGE('',*,*,#35854,.F.);
#50287=ORIENTED_EDGE('',*,*,#35995,.T.);
#50288=ORIENTED_EDGE('',*,*,#35996,.T.);
#50289=ORIENTED_EDGE('',*,*,#35852,.F.);
#50290=ORIENTED_EDGE('',*,*,#35997,.T.);
#50291=ORIENTED_EDGE('',*,*,#35758,.T.);
#50292=ORIENTED_EDGE('',*,*,#35851,.F.);
#50293=ORIENTED_EDGE('',*,*,#35998,.T.);
#50294=ORIENTED_EDGE('',*,*,#35759,.F.);
#50295=ORIENTED_EDGE('',*,*,#35997,.F.);
#50296=ORIENTED_EDGE('',*,*,#35850,.F.);
#50297=ORIENTED_EDGE('',*,*,#35999,.F.);
#50298=ORIENTED_EDGE('',*,*,#35760,.F.);
#50299=ORIENTED_EDGE('',*,*,#35998,.F.);
#50300=ORIENTED_EDGE('',*,*,#35848,.F.);
#50301=ORIENTED_EDGE('',*,*,#36000,.T.);
#50302=ORIENTED_EDGE('',*,*,#35762,.F.);
#50303=ORIENTED_EDGE('',*,*,#36001,.F.);
#50304=ORIENTED_EDGE('',*,*,#35847,.F.);
#50305=ORIENTED_EDGE('',*,*,#36002,.F.);
#50306=ORIENTED_EDGE('',*,*,#35763,.F.);
#50307=ORIENTED_EDGE('',*,*,#36000,.F.);
#50308=ORIENTED_EDGE('',*,*,#36002,.T.);
#50309=ORIENTED_EDGE('',*,*,#35846,.F.);
#50310=ORIENTED_EDGE('',*,*,#36003,.T.);
#50311=ORIENTED_EDGE('',*,*,#35764,.T.);
#50312=ORIENTED_EDGE('',*,*,#35999,.T.);
#50313=ORIENTED_EDGE('',*,*,#35849,.F.);
#50314=ORIENTED_EDGE('',*,*,#36001,.T.);
#50315=ORIENTED_EDGE('',*,*,#35761,.T.);
#50316=ORIENTED_EDGE('',*,*,#35766,.F.);
#50317=ORIENTED_EDGE('',*,*,#36004,.F.);
#50318=ORIENTED_EDGE('',*,*,#35844,.F.);
#50319=ORIENTED_EDGE('',*,*,#36005,.F.);
#50320=ORIENTED_EDGE('',*,*,#35765,.F.);
#50321=ORIENTED_EDGE('',*,*,#36003,.F.);
#50322=ORIENTED_EDGE('',*,*,#35845,.F.);
#50323=ORIENTED_EDGE('',*,*,#36004,.T.);
#50324=ORIENTED_EDGE('',*,*,#36005,.T.);
#50325=ORIENTED_EDGE('',*,*,#35843,.F.);
#50326=ORIENTED_EDGE('',*,*,#36006,.T.);
#50327=ORIENTED_EDGE('',*,*,#35767,.T.);
#50328=ORIENTED_EDGE('',*,*,#35842,.F.);
#50329=ORIENTED_EDGE('',*,*,#36007,.T.);
#50330=ORIENTED_EDGE('',*,*,#35768,.F.);
#50331=ORIENTED_EDGE('',*,*,#36006,.F.);
#50332=ORIENTED_EDGE('',*,*,#35841,.F.);
#50333=ORIENTED_EDGE('',*,*,#36008,.F.);
#50334=ORIENTED_EDGE('',*,*,#35769,.F.);
#50335=ORIENTED_EDGE('',*,*,#36007,.F.);
#50336=ORIENTED_EDGE('',*,*,#35839,.F.);
#50337=ORIENTED_EDGE('',*,*,#36009,.T.);
#50338=ORIENTED_EDGE('',*,*,#35771,.F.);
#50339=ORIENTED_EDGE('',*,*,#36010,.F.);
#50340=ORIENTED_EDGE('',*,*,#35838,.F.);
#50341=ORIENTED_EDGE('',*,*,#35776,.F.);
#50342=ORIENTED_EDGE('',*,*,#35772,.F.);
#50343=ORIENTED_EDGE('',*,*,#36009,.F.);
#50344=ORIENTED_EDGE('',*,*,#36011,.T.);
#50345=ORIENTED_EDGE('',*,*,#36012,.T.);
#50346=ORIENTED_EDGE('',*,*,#36013,.F.);
#50347=ORIENTED_EDGE('',*,*,#36012,.F.);
#50348=ORIENTED_EDGE('',*,*,#36014,.F.);
#50349=ORIENTED_EDGE('',*,*,#36013,.T.);
#50350=ORIENTED_EDGE('',*,*,#36015,.F.);
#50351=ORIENTED_EDGE('',*,*,#36016,.T.);
#50352=ORIENTED_EDGE('',*,*,#36014,.T.);
#50353=ORIENTED_EDGE('',*,*,#36016,.F.);
#50354=ORIENTED_EDGE('',*,*,#36017,.F.);
#50355=ORIENTED_EDGE('',*,*,#36018,.T.);
#50356=ORIENTED_EDGE('',*,*,#36015,.T.);
#50357=ORIENTED_EDGE('',*,*,#36018,.F.);
#50358=ORIENTED_EDGE('',*,*,#36019,.F.);
#50359=ORIENTED_EDGE('',*,*,#36020,.T.);
#50360=ORIENTED_EDGE('',*,*,#36017,.T.);
#50361=ORIENTED_EDGE('',*,*,#36020,.F.);
#50362=ORIENTED_EDGE('',*,*,#36021,.F.);
#50363=ORIENTED_EDGE('',*,*,#36019,.T.);
#50364=ORIENTED_EDGE('',*,*,#36022,.F.);
#50365=ORIENTED_EDGE('',*,*,#36023,.T.);
#50366=ORIENTED_EDGE('',*,*,#36021,.T.);
#50367=ORIENTED_EDGE('',*,*,#36023,.F.);
#50368=ORIENTED_EDGE('',*,*,#35639,.T.);
#50369=ORIENTED_EDGE('',*,*,#35641,.T.);
#50370=ORIENTED_EDGE('',*,*,#35640,.T.);
#50371=ORIENTED_EDGE('',*,*,#36024,.F.);
#50372=ORIENTED_EDGE('',*,*,#36025,.T.);
#50373=ORIENTED_EDGE('',*,*,#36022,.T.);
#50374=ORIENTED_EDGE('',*,*,#36025,.F.);
#50375=ORIENTED_EDGE('',*,*,#35711,.F.);
#50376=ORIENTED_EDGE('',*,*,#36024,.T.);
#50377=ORIENTED_EDGE('',*,*,#36008,.T.);
#50378=ORIENTED_EDGE('',*,*,#35840,.F.);
#50379=ORIENTED_EDGE('',*,*,#36010,.T.);
#50380=ORIENTED_EDGE('',*,*,#35770,.T.);
#50381=ORIENTED_EDGE('',*,*,#35784,.T.);
#50382=ORIENTED_EDGE('',*,*,#36026,.F.);
#50383=ORIENTED_EDGE('',*,*,#36026,.T.);
#50384=ORIENTED_EDGE('',*,*,#36027,.T.);
#50385=ORIENTED_EDGE('',*,*,#36028,.F.);
#50386=ORIENTED_EDGE('',*,*,#36027,.F.);
#50387=ORIENTED_EDGE('',*,*,#36028,.T.);
#50388=ORIENTED_EDGE('',*,*,#36029,.T.);
#50389=ORIENTED_EDGE('',*,*,#36030,.F.);
#50390=ORIENTED_EDGE('',*,*,#36029,.F.);
#50391=ORIENTED_EDGE('',*,*,#36030,.T.);
#50392=ORIENTED_EDGE('',*,*,#36031,.T.);
#50393=ORIENTED_EDGE('',*,*,#36011,.F.);
#50394=ORIENTED_EDGE('',*,*,#36031,.F.);
#50395=ORIENTED_EDGE('',*,*,#35645,.T.);
#50396=ORIENTED_EDGE('',*,*,#35646,.T.);
#50397=ORIENTED_EDGE('',*,*,#35643,.T.);
#50398=ORIENTED_EDGE('',*,*,#35636,.T.);
#59184=ADVANCED_FACE('',(#6084),#3096,.T.);
#59185=ADVANCED_FACE('',(#6085),#656,.F.);
#59186=ADVANCED_FACE('',(#6086),#3097,.T.);
#59187=ADVANCED_FACE('',(#6087),#3098,.F.);
#59188=ADVANCED_FACE('',(#6088),#3099,.F.);
#59189=ADVANCED_FACE('',(#6089),#914,.T.);
#59190=ADVANCED_FACE('',(#6090),#657,.T.);
#59191=ADVANCED_FACE('',(#6091),#658,.T.);
#59192=ADVANCED_FACE('',(#6092),#3100,.F.);
#59193=ADVANCED_FACE('',(#6093),#3101,.F.);
#59194=ADVANCED_FACE('',(#6094),#659,.T.);
#59195=ADVANCED_FACE('',(#6095),#915,.T.);
#59196=ADVANCED_FACE('',(#6096),#3102,.F.);
#59197=ADVANCED_FACE('',(#6097),#3103,.F.);
#59198=ADVANCED_FACE('',(#6098),#3104,.F.);
#59199=ADVANCED_FACE('',(#6099),#3105,.F.);
#59200=ADVANCED_FACE('',(#6100),#660,.T.);
#59201=ADVANCED_FACE('',(#6101),#661,.T.);
#59202=ADVANCED_FACE('',(#6102),#3106,.F.);
#59203=ADVANCED_FACE('',(#6103),#3107,.F.);
#59204=ADVANCED_FACE('',(#6104),#662,.T.);
#59205=ADVANCED_FACE('',(#6105),#3108,.F.);
#59206=ADVANCED_FACE('',(#6106),#3109,.F.);
#59207=ADVANCED_FACE('',(#6107),#3110,.F.);
#59208=ADVANCED_FACE('',(#6108),#3111,.F.);
#59209=ADVANCED_FACE('',(#6109),#663,.T.);
#59210=ADVANCED_FACE('',(#6110),#664,.T.);
#59211=ADVANCED_FACE('',(#6111),#3112,.F.);
#59212=ADVANCED_FACE('',(#6112),#3113,.F.);
#59213=ADVANCED_FACE('',(#6113),#665,.T.);
#59214=ADVANCED_FACE('',(#6114),#3114,.F.);
#59215=ADVANCED_FACE('',(#6115),#3115,.F.);
#59216=ADVANCED_FACE('',(#6116),#3116,.F.);
#59217=ADVANCED_FACE('',(#6117),#3117,.F.);
#59218=ADVANCED_FACE('',(#6118),#666,.T.);
#59219=ADVANCED_FACE('',(#6119),#667,.T.);
#59220=ADVANCED_FACE('',(#6120),#3118,.F.);
#59221=ADVANCED_FACE('',(#6121),#3119,.F.);
#59222=ADVANCED_FACE('',(#6122),#668,.T.);
#59223=ADVANCED_FACE('',(#6123),#3120,.F.);
#59224=ADVANCED_FACE('',(#6124),#3121,.F.);
#59225=ADVANCED_FACE('',(#6125),#3122,.F.);
#59226=ADVANCED_FACE('',(#6126),#3123,.F.);
#59227=ADVANCED_FACE('',(#6127),#669,.T.);
#59228=ADVANCED_FACE('',(#6128),#670,.T.);
#59229=ADVANCED_FACE('',(#6129),#3124,.F.);
#59230=ADVANCED_FACE('',(#6130),#3125,.F.);
#59231=ADVANCED_FACE('',(#6131),#671,.T.);
#59232=ADVANCED_FACE('',(#6132),#3126,.F.);
#59233=ADVANCED_FACE('',(#6133),#3127,.F.);
#59234=ADVANCED_FACE('',(#6134),#3128,.F.);
#59235=ADVANCED_FACE('',(#6135),#3129,.F.);
#59236=ADVANCED_FACE('',(#6136),#672,.T.);
#59237=ADVANCED_FACE('',(#6137),#673,.T.);
#59238=ADVANCED_FACE('',(#6138),#3130,.F.);
#59239=ADVANCED_FACE('',(#6139),#3131,.F.);
#59240=ADVANCED_FACE('',(#6140),#674,.T.);
#59241=ADVANCED_FACE('',(#6141),#3132,.F.);
#59242=ADVANCED_FACE('',(#6142),#3133,.F.);
#59243=ADVANCED_FACE('',(#6143),#3134,.F.);
#59244=ADVANCED_FACE('',(#6144),#3135,.F.);
#59245=ADVANCED_FACE('',(#6145),#675,.T.);
#59246=ADVANCED_FACE('',(#6146),#676,.T.);
#59247=ADVANCED_FACE('',(#6147),#3136,.F.);
#59248=ADVANCED_FACE('',(#6148),#3137,.F.);
#59249=ADVANCED_FACE('',(#6149),#677,.T.);
#59250=ADVANCED_FACE('',(#6150),#3138,.F.);
#59251=ADVANCED_FACE('',(#6151),#3139,.F.);
#59252=ADVANCED_FACE('',(#6152),#3140,.F.);
#59253=ADVANCED_FACE('',(#6153),#3141,.F.);
#59254=ADVANCED_FACE('',(#6154),#678,.T.);
#59255=ADVANCED_FACE('',(#6155),#679,.T.);
#59256=ADVANCED_FACE('',(#6156),#3142,.F.);
#59257=ADVANCED_FACE('',(#6157),#3143,.F.);
#59258=ADVANCED_FACE('',(#6158),#680,.T.);
#59259=ADVANCED_FACE('',(#6159),#3144,.F.);
#59260=ADVANCED_FACE('',(#6160),#3145,.F.);
#59261=ADVANCED_FACE('',(#6161),#3146,.F.);
#59262=ADVANCED_FACE('',(#6162),#3147,.F.);
#59263=ADVANCED_FACE('',(#6163),#681,.T.);
#59264=ADVANCED_FACE('',(#6164),#682,.T.);
#59265=ADVANCED_FACE('',(#6165),#3148,.F.);
#59266=ADVANCED_FACE('',(#6166),#3149,.F.);
#59267=ADVANCED_FACE('',(#6167),#683,.T.);
#59268=ADVANCED_FACE('',(#6168),#3150,.F.);
#59269=ADVANCED_FACE('',(#6169),#3151,.F.);
#59270=ADVANCED_FACE('',(#6170),#3152,.F.);
#59271=ADVANCED_FACE('',(#6171),#3153,.F.);
#59272=ADVANCED_FACE('',(#6172),#684,.T.);
#59273=ADVANCED_FACE('',(#6173),#685,.T.);
#59274=ADVANCED_FACE('',(#6174),#3154,.F.);
#59275=ADVANCED_FACE('',(#6175),#3155,.F.);
#59276=ADVANCED_FACE('',(#6176),#686,.T.);
#59277=ADVANCED_FACE('',(#6177),#3156,.F.);
#59278=ADVANCED_FACE('',(#6178),#3157,.F.);
#59279=ADVANCED_FACE('',(#6179),#3158,.F.);
#59280=ADVANCED_FACE('',(#6180),#3159,.F.);
#59281=ADVANCED_FACE('',(#6181),#687,.T.);
#59282=ADVANCED_FACE('',(#6182),#688,.T.);
#59283=ADVANCED_FACE('',(#6183),#3160,.F.);
#59284=ADVANCED_FACE('',(#6184),#3161,.F.);
#59285=ADVANCED_FACE('',(#6185),#689,.T.);
#59286=ADVANCED_FACE('',(#6186),#3162,.F.);
#59287=ADVANCED_FACE('',(#6187),#3163,.F.);
#59288=ADVANCED_FACE('',(#6188),#3164,.F.);
#59289=ADVANCED_FACE('',(#6189),#3165,.F.);
#59290=ADVANCED_FACE('',(#6190),#690,.T.);
#59291=ADVANCED_FACE('',(#6191),#691,.T.);
#59292=ADVANCED_FACE('',(#6192),#3166,.F.);
#59293=ADVANCED_FACE('',(#6193),#3167,.F.);
#59294=ADVANCED_FACE('',(#6194),#692,.T.);
#59295=ADVANCED_FACE('',(#6195),#3168,.F.);
#59296=ADVANCED_FACE('',(#6196),#3169,.F.);
#59297=ADVANCED_FACE('',(#6197),#3170,.F.);
#59298=ADVANCED_FACE('',(#6198),#3171,.F.);
#59299=ADVANCED_FACE('',(#6199),#693,.T.);
#59300=ADVANCED_FACE('',(#6200),#694,.T.);
#59301=ADVANCED_FACE('',(#6201),#3172,.F.);
#59302=ADVANCED_FACE('',(#6202),#3173,.F.);
#59303=ADVANCED_FACE('',(#6203),#695,.T.);
#59304=ADVANCED_FACE('',(#6204),#3174,.F.);
#59305=ADVANCED_FACE('',(#6205),#3175,.F.);
#59306=ADVANCED_FACE('',(#6206),#3176,.F.);
#59307=ADVANCED_FACE('',(#6207),#3177,.F.);
#59308=ADVANCED_FACE('',(#6208),#916,.F.);
#59309=ADVANCED_FACE('',(#6209,#1832),#3178,.T.);
#59310=ADVANCED_FACE('',(#6210),#917,.T.);
#59311=ADVANCED_FACE('',(#6211),#696,.T.);
#59312=ADVANCED_FACE('',(#6212),#918,.T.);
#59313=ADVANCED_FACE('',(#6213,#1833),#3179,.T.);
#59314=ADVANCED_FACE('',(#6214,#1834),#697,.T.);
#59315=ADVANCED_FACE('',(#6215),#919,.T.);
#59316=ADVANCED_FACE('',(#6216,#1835),#3180,.T.);
#59317=ADVANCED_FACE('',(#6217),#698,.T.);
#59318=ADVANCED_FACE('',(#6218,#1836),#3181,.T.);
#59319=ADVANCED_FACE('',(#6219),#920,.F.);
#59320=ADVANCED_FACE('',(#6220),#3182,.T.);
#59321=ADVANCED_FACE('',(#6221),#921,.F.);
#59322=ADVANCED_FACE('',(#6222,#1837),#699,.F.);
#60397=CLOSED_SHELL('',(#59184,#59185,#59186,#59187,#59188,#59189,#59190,
#59191,#59192,#59193,#59194,#59195,#59196,#59197,#59198,#59199,#59200,#59201,
#59202,#59203,#59204,#59205,#59206,#59207,#59208,#59209,#59210,#59211,#59212,
#59213,#59214,#59215,#59216,#59217,#59218,#59219,#59220,#59221,#59222,#59223,
#59224,#59225,#59226,#59227,#59228,#59229,#59230,#59231,#59232,#59233,#59234,
#59235,#59236,#59237,#59238,#59239,#59240,#59241,#59242,#59243,#59244,#59245,
#59246,#59247,#59248,#59249,#59250,#59251,#59252,#59253,#59254,#59255,#59256,
#59257,#59258,#59259,#59260,#59261,#59262,#59263,#59264,#59265,#59266,#59267,
#59268,#59269,#59270,#59271,#59272,#59273,#59274,#59275,#59276,#59277,#59278,
#59279,#59280,#59281,#59282,#59283,#59284,#59285,#59286,#59287,#59288,#59289,
#59290,#59291,#59292,#59293,#59294,#59295,#59296,#59297,#59298,#59299,#59300,
#59301,#59302,#59303,#59304,#59305,#59306,#59307,#59308,#59309,#59310,#59311,
#59312,#59313,#59314,#59315,#59316,#59317,#59318,#59319,#59320,#59321,#59322));
#62138=AXIS2_PLACEMENT_3D('',#97718,#70454,#70455);
#62139=AXIS2_PLACEMENT_3D('',#97719,#70456,#70457);
#62140=AXIS2_PLACEMENT_3D('',#97724,#70459,#70460);
#62141=AXIS2_PLACEMENT_3D('',#97725,#70461,#70462);
#62142=AXIS2_PLACEMENT_3D('',#97726,#70463,#70464);
#62143=AXIS2_PLACEMENT_3D('',#97790,#70466,#70467);
#62144=AXIS2_PLACEMENT_3D('',#97809,#70468,#70469);
#62145=AXIS2_PLACEMENT_3D('',#97811,#70471,#70472);
#62146=AXIS2_PLACEMENT_3D('',#97824,#70475,#70476);
#62147=AXIS2_PLACEMENT_3D('',#97834,#70478,#70479);
#62148=AXIS2_PLACEMENT_3D('',#97836,#70480,#70481);
#62149=AXIS2_PLACEMENT_3D('',#97846,#70482,#70483);
#62150=AXIS2_PLACEMENT_3D('',#97856,#70484,#70485);
#62151=AXIS2_PLACEMENT_3D('',#97866,#70486,#70487);
#62152=AXIS2_PLACEMENT_3D('',#97876,#70488,#70489);
#62153=AXIS2_PLACEMENT_3D('',#97886,#70490,#70491);
#62154=AXIS2_PLACEMENT_3D('',#97896,#70492,#70493);
#62155=AXIS2_PLACEMENT_3D('',#97906,#70494,#70495);
#62156=AXIS2_PLACEMENT_3D('',#97916,#70496,#70497);
#62157=AXIS2_PLACEMENT_3D('',#97926,#70498,#70499);
#62158=AXIS2_PLACEMENT_3D('',#97936,#70500,#70501);
#62159=AXIS2_PLACEMENT_3D('',#97946,#70502,#70503);
#62160=AXIS2_PLACEMENT_3D('',#97956,#70504,#70505);
#62161=AXIS2_PLACEMENT_3D('',#97966,#70506,#70507);
#62162=AXIS2_PLACEMENT_3D('',#97976,#70508,#70509);
#62163=AXIS2_PLACEMENT_3D('',#97986,#70510,#70511);
#62164=AXIS2_PLACEMENT_3D('',#97996,#70512,#70513);
#62165=AXIS2_PLACEMENT_3D('',#98006,#70514,#70515);
#62166=AXIS2_PLACEMENT_3D('',#98016,#70516,#70517);
#62167=AXIS2_PLACEMENT_3D('',#98023,#70519,#70520);
#62168=AXIS2_PLACEMENT_3D('',#98029,#70521,#70522);
#62169=AXIS2_PLACEMENT_3D('',#98039,#70523,#70524);
#62170=AXIS2_PLACEMENT_3D('',#98049,#70525,#70526);
#62171=AXIS2_PLACEMENT_3D('',#98059,#70527,#70528);
#62172=AXIS2_PLACEMENT_3D('',#98069,#70529,#70530);
#62173=AXIS2_PLACEMENT_3D('',#98079,#70531,#70532);
#62174=AXIS2_PLACEMENT_3D('',#98089,#70533,#70534);
#62175=AXIS2_PLACEMENT_3D('',#98099,#70535,#70536);
#62176=AXIS2_PLACEMENT_3D('',#98109,#70537,#70538);
#62177=AXIS2_PLACEMENT_3D('',#98119,#70539,#70540);
#62178=AXIS2_PLACEMENT_3D('',#98129,#70541,#70542);
#62179=AXIS2_PLACEMENT_3D('',#98139,#70543,#70544);
#62180=AXIS2_PLACEMENT_3D('',#98149,#70545,#70546);
#62181=AXIS2_PLACEMENT_3D('',#98159,#70547,#70548);
#62182=AXIS2_PLACEMENT_3D('',#98169,#70549,#70550);
#62183=AXIS2_PLACEMENT_3D('',#98179,#70551,#70552);
#62184=AXIS2_PLACEMENT_3D('',#98189,#70553,#70554);
#62185=AXIS2_PLACEMENT_3D('',#98199,#70555,#70556);
#62186=AXIS2_PLACEMENT_3D('',#98209,#70557,#70558);
#62187=AXIS2_PLACEMENT_3D('',#98219,#70559,#70560);
#62188=AXIS2_PLACEMENT_3D('',#98228,#70561,#70562);
#62189=AXIS2_PLACEMENT_3D('',#98229,#70563,#70564);
#62190=AXIS2_PLACEMENT_3D('',#98231,#70565,#70566);
#62191=AXIS2_PLACEMENT_3D('',#98233,#70568,#70569);
#62192=AXIS2_PLACEMENT_3D('',#98236,#70571,#70572);
#62193=AXIS2_PLACEMENT_3D('',#98237,#70573,#70574);
#62194=AXIS2_PLACEMENT_3D('',#98245,#70577,#70578);
#62195=AXIS2_PLACEMENT_3D('',#98249,#70579,#70580);
#62196=AXIS2_PLACEMENT_3D('',#98251,#70581,#70582);
#62197=AXIS2_PLACEMENT_3D('',#98253,#70584,#70585);
#62198=AXIS2_PLACEMENT_3D('',#98255,#70586,#70587);
#62199=AXIS2_PLACEMENT_3D('',#98263,#70589,#70590);
#62200=AXIS2_PLACEMENT_3D('',#98273,#70591,#70592);
#62201=AXIS2_PLACEMENT_3D('',#98283,#70593,#70594);
#62202=AXIS2_PLACEMENT_3D('',#98293,#70595,#70596);
#62203=AXIS2_PLACEMENT_3D('',#98303,#70597,#70598);
#62204=AXIS2_PLACEMENT_3D('',#98313,#70599,#70600);
#62205=AXIS2_PLACEMENT_3D('',#98323,#70601,#70602);
#62206=AXIS2_PLACEMENT_3D('',#98333,#70603,#70604);
#62207=AXIS2_PLACEMENT_3D('',#98343,#70605,#70606);
#62208=AXIS2_PLACEMENT_3D('',#98353,#70607,#70608);
#62209=AXIS2_PLACEMENT_3D('',#98363,#70609,#70610);
#62210=AXIS2_PLACEMENT_3D('',#98373,#70611,#70612);
#62211=AXIS2_PLACEMENT_3D('',#98383,#70613,#70614);
#62212=AXIS2_PLACEMENT_3D('',#98393,#70615,#70616);
#62213=AXIS2_PLACEMENT_3D('',#98403,#70617,#70618);
#62214=AXIS2_PLACEMENT_3D('',#98413,#70619,#70620);
#62215=AXIS2_PLACEMENT_3D('',#98423,#70621,#70622);
#62216=AXIS2_PLACEMENT_3D('',#98440,#70623,#70624);
#62217=AXIS2_PLACEMENT_3D('',#98450,#70625,#70626);
#62218=AXIS2_PLACEMENT_3D('',#98460,#70627,#70628);
#62219=AXIS2_PLACEMENT_3D('',#98470,#70629,#70630);
#62220=AXIS2_PLACEMENT_3D('',#98480,#70631,#70632);
#62221=AXIS2_PLACEMENT_3D('',#98490,#70633,#70634);
#62222=AXIS2_PLACEMENT_3D('',#98500,#70635,#70636);
#62223=AXIS2_PLACEMENT_3D('',#98510,#70637,#70638);
#62224=AXIS2_PLACEMENT_3D('',#98520,#70639,#70640);
#62225=AXIS2_PLACEMENT_3D('',#98530,#70641,#70642);
#62226=AXIS2_PLACEMENT_3D('',#98540,#70643,#70644);
#62227=AXIS2_PLACEMENT_3D('',#98550,#70645,#70646);
#62228=AXIS2_PLACEMENT_3D('',#98560,#70647,#70648);
#62229=AXIS2_PLACEMENT_3D('',#98570,#70649,#70650);
#62230=AXIS2_PLACEMENT_3D('',#98580,#70651,#70652);
#62231=AXIS2_PLACEMENT_3D('',#98590,#70653,#70654);
#62232=AXIS2_PLACEMENT_3D('',#98600,#70655,#70656);
#62233=AXIS2_PLACEMENT_3D('',#98610,#70657,#70658);
#62234=AXIS2_PLACEMENT_3D('',#98620,#70659,#70660);
#62235=AXIS2_PLACEMENT_3D('',#98630,#70661,#70662);
#62236=AXIS2_PLACEMENT_3D('',#98634,#70663,#70664);
#62237=AXIS2_PLACEMENT_3D('',#98636,#70666,#70667);
#62238=AXIS2_PLACEMENT_3D('',#98638,#70669,#70670);
#62239=AXIS2_PLACEMENT_3D('',#98641,#70673,#70674);
#62240=AXIS2_PLACEMENT_3D('',#98643,#70676,#70677);
#62241=AXIS2_PLACEMENT_3D('',#98645,#70679,#70680);
#62242=AXIS2_PLACEMENT_3D('',#98646,#70681,#70682);
#62243=AXIS2_PLACEMENT_3D('',#98649,#70685,#70686);
#62244=AXIS2_PLACEMENT_3D('',#98650,#70687,#70688);
#62245=AXIS2_PLACEMENT_3D('',#98652,#70690,#70691);
#62246=AXIS2_PLACEMENT_3D('',#98654,#70693,#70694);
#62247=AXIS2_PLACEMENT_3D('',#98656,#70696,#70697);
#62248=AXIS2_PLACEMENT_3D('',#98659,#70700,#70701);
#62249=AXIS2_PLACEMENT_3D('',#98661,#70703,#70704);
#62250=AXIS2_PLACEMENT_3D('',#98663,#70706,#70707);
#62251=AXIS2_PLACEMENT_3D('',#98664,#70708,#70709);
#62252=AXIS2_PLACEMENT_3D('',#98667,#70712,#70713);
#62253=AXIS2_PLACEMENT_3D('',#98668,#70714,#70715);
#62254=AXIS2_PLACEMENT_3D('',#98670,#70717,#70718);
#62255=AXIS2_PLACEMENT_3D('',#98672,#70720,#70721);
#62256=AXIS2_PLACEMENT_3D('',#98674,#70723,#70724);
#62257=AXIS2_PLACEMENT_3D('',#98677,#70727,#70728);
#62258=AXIS2_PLACEMENT_3D('',#98679,#70730,#70731);
#62259=AXIS2_PLACEMENT_3D('',#98681,#70733,#70734);
#62260=AXIS2_PLACEMENT_3D('',#98682,#70735,#70736);
#62261=AXIS2_PLACEMENT_3D('',#98685,#70739,#70740);
#62262=AXIS2_PLACEMENT_3D('',#98686,#70741,#70742);
#62263=AXIS2_PLACEMENT_3D('',#98688,#70744,#70745);
#62264=AXIS2_PLACEMENT_3D('',#98690,#70747,#70748);
#62265=AXIS2_PLACEMENT_3D('',#98692,#70750,#70751);
#62266=AXIS2_PLACEMENT_3D('',#98695,#70754,#70755);
#62267=AXIS2_PLACEMENT_3D('',#98697,#70757,#70758);
#62268=AXIS2_PLACEMENT_3D('',#98699,#70760,#70761);
#62269=AXIS2_PLACEMENT_3D('',#98700,#70762,#70763);
#62270=AXIS2_PLACEMENT_3D('',#98703,#70766,#70767);
#62271=AXIS2_PLACEMENT_3D('',#98704,#70768,#70769);
#62272=AXIS2_PLACEMENT_3D('',#98706,#70771,#70772);
#62273=AXIS2_PLACEMENT_3D('',#98708,#70774,#70775);
#62274=AXIS2_PLACEMENT_3D('',#98710,#70777,#70778);
#62275=AXIS2_PLACEMENT_3D('',#98713,#70781,#70782);
#62276=AXIS2_PLACEMENT_3D('',#98715,#70784,#70785);
#62277=AXIS2_PLACEMENT_3D('',#98717,#70787,#70788);
#62278=AXIS2_PLACEMENT_3D('',#98718,#70789,#70790);
#62279=AXIS2_PLACEMENT_3D('',#98721,#70793,#70794);
#62280=AXIS2_PLACEMENT_3D('',#98722,#70795,#70796);
#62281=AXIS2_PLACEMENT_3D('',#98724,#70798,#70799);
#62282=AXIS2_PLACEMENT_3D('',#98726,#70801,#70802);
#62283=AXIS2_PLACEMENT_3D('',#98728,#70804,#70805);
#62284=AXIS2_PLACEMENT_3D('',#98731,#70808,#70809);
#62285=AXIS2_PLACEMENT_3D('',#98733,#70811,#70812);
#62286=AXIS2_PLACEMENT_3D('',#98735,#70814,#70815);
#62287=AXIS2_PLACEMENT_3D('',#98736,#70816,#70817);
#62288=AXIS2_PLACEMENT_3D('',#98739,#70820,#70821);
#62289=AXIS2_PLACEMENT_3D('',#98740,#70822,#70823);
#62290=AXIS2_PLACEMENT_3D('',#98742,#70825,#70826);
#62291=AXIS2_PLACEMENT_3D('',#98744,#70828,#70829);
#62292=AXIS2_PLACEMENT_3D('',#98746,#70831,#70832);
#62293=AXIS2_PLACEMENT_3D('',#98749,#70835,#70836);
#62294=AXIS2_PLACEMENT_3D('',#98751,#70838,#70839);
#62295=AXIS2_PLACEMENT_3D('',#98753,#70841,#70842);
#62296=AXIS2_PLACEMENT_3D('',#98754,#70843,#70844);
#62297=AXIS2_PLACEMENT_3D('',#98757,#70847,#70848);
#62298=AXIS2_PLACEMENT_3D('',#98758,#70849,#70850);
#62299=AXIS2_PLACEMENT_3D('',#98760,#70852,#70853);
#62300=AXIS2_PLACEMENT_3D('',#98762,#70855,#70856);
#62301=AXIS2_PLACEMENT_3D('',#98764,#70858,#70859);
#62302=AXIS2_PLACEMENT_3D('',#98767,#70862,#70863);
#62303=AXIS2_PLACEMENT_3D('',#98769,#70865,#70866);
#62304=AXIS2_PLACEMENT_3D('',#98771,#70868,#70869);
#62305=AXIS2_PLACEMENT_3D('',#98772,#70870,#70871);
#62306=AXIS2_PLACEMENT_3D('',#98775,#70874,#70875);
#62307=AXIS2_PLACEMENT_3D('',#98776,#70876,#70877);
#62308=AXIS2_PLACEMENT_3D('',#98778,#70879,#70880);
#62309=AXIS2_PLACEMENT_3D('',#98780,#70882,#70883);
#62310=AXIS2_PLACEMENT_3D('',#98782,#70885,#70886);
#62311=AXIS2_PLACEMENT_3D('',#98785,#70889,#70890);
#62312=AXIS2_PLACEMENT_3D('',#98787,#70892,#70893);
#62313=AXIS2_PLACEMENT_3D('',#98789,#70895,#70896);
#62314=AXIS2_PLACEMENT_3D('',#98790,#70897,#70898);
#62315=AXIS2_PLACEMENT_3D('',#98793,#70901,#70902);
#62316=AXIS2_PLACEMENT_3D('',#98794,#70903,#70904);
#62317=AXIS2_PLACEMENT_3D('',#98796,#70906,#70907);
#62318=AXIS2_PLACEMENT_3D('',#98798,#70909,#70910);
#62319=AXIS2_PLACEMENT_3D('',#98800,#70912,#70913);
#62320=AXIS2_PLACEMENT_3D('',#98803,#70916,#70917);
#62321=AXIS2_PLACEMENT_3D('',#98805,#70919,#70920);
#62322=AXIS2_PLACEMENT_3D('',#98807,#70922,#70923);
#62323=AXIS2_PLACEMENT_3D('',#98808,#70924,#70925);
#62324=AXIS2_PLACEMENT_3D('',#98811,#70928,#70929);
#62325=AXIS2_PLACEMENT_3D('',#98812,#70930,#70931);
#62326=AXIS2_PLACEMENT_3D('',#98814,#70933,#70934);
#62327=AXIS2_PLACEMENT_3D('',#98816,#70936,#70937);
#62328=AXIS2_PLACEMENT_3D('',#98818,#70939,#70940);
#62329=AXIS2_PLACEMENT_3D('',#98821,#70943,#70944);
#62330=AXIS2_PLACEMENT_3D('',#98823,#70946,#70947);
#62331=AXIS2_PLACEMENT_3D('',#98825,#70949,#70950);
#62332=AXIS2_PLACEMENT_3D('',#98826,#70951,#70952);
#62333=AXIS2_PLACEMENT_3D('',#98829,#70955,#70956);
#62334=AXIS2_PLACEMENT_3D('',#98830,#70957,#70958);
#62335=AXIS2_PLACEMENT_3D('',#98832,#70960,#70961);
#62336=AXIS2_PLACEMENT_3D('',#98834,#70963,#70964);
#62337=AXIS2_PLACEMENT_3D('',#98836,#70966,#70967);
#62338=AXIS2_PLACEMENT_3D('',#98839,#70970,#70971);
#62339=AXIS2_PLACEMENT_3D('',#98841,#70973,#70974);
#62340=AXIS2_PLACEMENT_3D('',#98843,#70976,#70977);
#62341=AXIS2_PLACEMENT_3D('',#98844,#70978,#70979);
#62342=AXIS2_PLACEMENT_3D('',#98847,#70982,#70983);
#62343=AXIS2_PLACEMENT_3D('',#98848,#70984,#70985);
#62344=AXIS2_PLACEMENT_3D('',#98850,#70987,#70988);
#62345=AXIS2_PLACEMENT_3D('',#98852,#70990,#70991);
#62346=AXIS2_PLACEMENT_3D('',#98854,#70993,#70994);
#62347=AXIS2_PLACEMENT_3D('',#98857,#70997,#70998);
#62348=AXIS2_PLACEMENT_3D('',#98858,#70999,#71000);
#62349=AXIS2_PLACEMENT_3D('',#98860,#71001,#71002);
#62350=AXIS2_PLACEMENT_3D('',#98863,#71004,#71005);
#62351=AXIS2_PLACEMENT_3D('',#98864,#71006,#71007);
#62352=AXIS2_PLACEMENT_3D('',#98866,#71008,#71009);
#62353=AXIS2_PLACEMENT_3D('',#98867,#71010,#71011);
#62354=AXIS2_PLACEMENT_3D('',#98869,#71012,#71013);
#62355=AXIS2_PLACEMENT_3D('',#98871,#71015,#71016);
#62356=AXIS2_PLACEMENT_3D('',#98873,#71017,#71018);
#62357=AXIS2_PLACEMENT_3D('',#98875,#71020,#71021);
#62358=AXIS2_PLACEMENT_3D('',#98877,#71022,#71023);
#62359=AXIS2_PLACEMENT_3D('',#98879,#71025,#71026);
#62360=AXIS2_PLACEMENT_3D('',#98881,#71027,#71028);
#62361=AXIS2_PLACEMENT_3D('',#98882,#71029,#71030);
#62362=AXIS2_PLACEMENT_3D('',#98884,#71031,#71032);
#62363=AXIS2_PLACEMENT_3D('',#98886,#71034,#71035);
#62364=AXIS2_PLACEMENT_3D('',#98888,#71036,#71037);
#62365=AXIS2_PLACEMENT_3D('',#98890,#71039,#71040);
#62366=AXIS2_PLACEMENT_3D('',#98891,#71041,#71042);
#62367=AXIS2_PLACEMENT_3D('',#98892,#71043,#71044);
#62368=AXIS2_PLACEMENT_3D('',#98894,#71045,#71046);
#62369=AXIS2_PLACEMENT_3D('',#98895,#71047,#71048);
#62370=AXIS2_PLACEMENT_3D('',#98898,#71050,#71051);
#62371=AXIS2_PLACEMENT_3D('',#98899,#71052,#71053);
#62372=AXIS2_PLACEMENT_3D('',#98900,#71054,#71055);
#62373=AXIS2_PLACEMENT_3D('',#98904,#71057,#71058);
#62374=AXIS2_PLACEMENT_3D('',#98905,#71059,#71060);
#70454=DIRECTION('axis',(0.,0.,1.));
#70455=DIRECTION('refdir',(1.,0.,0.));
#70456=DIRECTION('center_axis',(0.,1.,0.));
#70457=DIRECTION('ref_axis',(1.,0.,0.));
#70458=DIRECTION('',(0.,0.,1.));
#70459=DIRECTION('center_axis',(0.,-1.,0.));
#70460=DIRECTION('ref_axis',(1.,0.,0.));
#70461=DIRECTION('center_axis',(0.,-1.,0.));
#70462=DIRECTION('ref_axis',(1.,0.,0.));
#70463=DIRECTION('center_axis',(0.,-1.,0.));
#70464=DIRECTION('ref_axis',(1.,0.,0.));
#70465=DIRECTION('',(0.,-1.,0.));
#70466=DIRECTION('center_axis',(0.,-1.,0.));
#70467=DIRECTION('ref_axis',(1.,0.,0.));
#70468=DIRECTION('center_axis',(0.,1.,0.));
#70469=DIRECTION('ref_axis',(1.,0.,0.));
#70470=DIRECTION('',(0.,0.,-1.));
#70471=DIRECTION('center_axis',(-0.402510663229762,0.915415297002588,0.));
#70472=DIRECTION('ref_axis',(0.915415297002588,0.402510663229762,0.));
#70473=DIRECTION('',(0.,0.,-1.));
#70474=DIRECTION('',(0.,0.,-1.));
#70475=DIRECTION('center_axis',(-0.66568927282754,-0.746229047975447,0.));
#70476=DIRECTION('ref_axis',(-0.746229047975447,0.66568927282754,0.));
#70477=DIRECTION('',(0.,0.,1.));
#70478=DIRECTION('center_axis',(0.,0.,1.));
#70479=DIRECTION('ref_axis',(1.,0.,0.));
#70480=DIRECTION('center_axis',(0.,0.,1.));
#70481=DIRECTION('ref_axis',(1.,0.,0.));
#70482=DIRECTION('center_axis',(0.,0.,1.));
#70483=DIRECTION('ref_axis',(1.,0.,0.));
#70484=DIRECTION('center_axis',(0.,0.,1.));
#70485=DIRECTION('ref_axis',(1.,0.,0.));
#70486=DIRECTION('center_axis',(0.,0.,1.));
#70487=DIRECTION('ref_axis',(1.,0.,0.));
#70488=DIRECTION('center_axis',(0.,0.,1.));
#70489=DIRECTION('ref_axis',(1.,0.,0.));
#70490=DIRECTION('center_axis',(0.,0.,1.));
#70491=DIRECTION('ref_axis',(1.,0.,0.));
#70492=DIRECTION('center_axis',(0.,0.,1.));
#70493=DIRECTION('ref_axis',(1.,0.,0.));
#70494=DIRECTION('center_axis',(0.,0.,1.));
#70495=DIRECTION('ref_axis',(1.,0.,0.));
#70496=DIRECTION('center_axis',(0.,0.,1.));
#70497=DIRECTION('ref_axis',(1.,0.,0.));
#70498=DIRECTION('center_axis',(0.,0.,1.));
#70499=DIRECTION('ref_axis',(1.,0.,0.));
#70500=DIRECTION('center_axis',(0.,0.,1.));
#70501=DIRECTION('ref_axis',(1.,0.,0.));
#70502=DIRECTION('center_axis',(0.,0.,1.));
#70503=DIRECTION('ref_axis',(1.,0.,0.));
#70504=DIRECTION('center_axis',(0.,0.,1.));
#70505=DIRECTION('ref_axis',(1.,0.,0.));
#70506=DIRECTION('center_axis',(0.,0.,1.));
#70507=DIRECTION('ref_axis',(1.,0.,0.));
#70508=DIRECTION('center_axis',(0.,0.,1.));
#70509=DIRECTION('ref_axis',(1.,0.,0.));
#70510=DIRECTION('center_axis',(0.,0.,1.));
#70511=DIRECTION('ref_axis',(1.,0.,0.));
#70512=DIRECTION('center_axis',(0.,0.,1.));
#70513=DIRECTION('ref_axis',(1.,0.,0.));
#70514=DIRECTION('center_axis',(0.,0.,1.));
#70515=DIRECTION('ref_axis',(1.,0.,0.));
#70516=DIRECTION('center_axis',(0.,0.,1.));
#70517=DIRECTION('ref_axis',(1.,0.,0.));
#70518=DIRECTION('',(0.707106781186547,8.65956056235493E-17,-0.707106781186547));
#70519=DIRECTION('center_axis',(0.,0.,1.));
#70520=DIRECTION('ref_axis',(1.,0.,0.));
#70521=DIRECTION('center_axis',(0.,0.,1.));
#70522=DIRECTION('ref_axis',(1.,0.,0.));
#70523=DIRECTION('center_axis',(0.,0.,1.));
#70524=DIRECTION('ref_axis',(1.,0.,0.));
#70525=DIRECTION('center_axis',(0.,0.,1.));
#70526=DIRECTION('ref_axis',(1.,0.,0.));
#70527=DIRECTION('center_axis',(0.,0.,1.));
#70528=DIRECTION('ref_axis',(1.,0.,0.));
#70529=DIRECTION('center_axis',(0.,0.,1.));
#70530=DIRECTION('ref_axis',(1.,0.,0.));
#70531=DIRECTION('center_axis',(0.,0.,1.));
#70532=DIRECTION('ref_axis',(1.,0.,0.));
#70533=DIRECTION('center_axis',(0.,0.,1.));
#70534=DIRECTION('ref_axis',(1.,0.,0.));
#70535=DIRECTION('center_axis',(0.,0.,1.));
#70536=DIRECTION('ref_axis',(1.,0.,0.));
#70537=DIRECTION('center_axis',(0.,0.,1.));
#70538=DIRECTION('ref_axis',(1.,0.,0.));
#70539=DIRECTION('center_axis',(0.,0.,1.));
#70540=DIRECTION('ref_axis',(1.,0.,0.));
#70541=DIRECTION('center_axis',(0.,0.,1.));
#70542=DIRECTION('ref_axis',(1.,0.,0.));
#70543=DIRECTION('center_axis',(0.,0.,1.));
#70544=DIRECTION('ref_axis',(1.,0.,0.));
#70545=DIRECTION('center_axis',(0.,0.,1.));
#70546=DIRECTION('ref_axis',(1.,0.,0.));
#70547=DIRECTION('center_axis',(0.,0.,1.));
#70548=DIRECTION('ref_axis',(1.,0.,0.));
#70549=DIRECTION('center_axis',(0.,0.,1.));
#70550=DIRECTION('ref_axis',(1.,0.,0.));
#70551=DIRECTION('center_axis',(0.,0.,1.));
#70552=DIRECTION('ref_axis',(1.,0.,0.));
#70553=DIRECTION('center_axis',(0.,0.,1.));
#70554=DIRECTION('ref_axis',(1.,0.,0.));
#70555=DIRECTION('center_axis',(0.,0.,1.));
#70556=DIRECTION('ref_axis',(1.,0.,0.));
#70557=DIRECTION('center_axis',(0.,0.,1.));
#70558=DIRECTION('ref_axis',(1.,0.,0.));
#70559=DIRECTION('center_axis',(0.,0.,1.));
#70560=DIRECTION('ref_axis',(1.,0.,0.));
#70561=DIRECTION('center_axis',(0.,0.,1.));
#70562=DIRECTION('ref_axis',(1.,0.,0.));
#70563=DIRECTION('center_axis',(0.,0.,1.));
#70564=DIRECTION('ref_axis',(1.,0.,0.));
#70565=DIRECTION('center_axis',(0.,0.,1.));
#70566=DIRECTION('ref_axis',(1.,0.,0.));
#70567=DIRECTION('',(0.,0.,-1.));
#70568=DIRECTION('center_axis',(0.,0.,1.));
#70569=DIRECTION('ref_axis',(1.,0.,0.));
#70570=DIRECTION('',(0.,0.,1.));
#70571=DIRECTION('center_axis',(0.,0.,1.));
#70572=DIRECTION('ref_axis',(1.,0.,0.));
#70573=DIRECTION('center_axis',(-0.774229475148536,-0.632904984820962,0.));
#70574=DIRECTION('ref_axis',(-0.632904984820962,0.774229475148536,0.));
#70575=DIRECTION('',(0.,0.,-1.));
#70576=DIRECTION('',(0.,0.,1.));
#70577=DIRECTION('center_axis',(-0.254352586761008,0.967111555927228,0.));
#70578=DIRECTION('ref_axis',(0.967111555927228,0.254352586761008,0.));
#70579=DIRECTION('center_axis',(0.,0.,1.));
#70580=DIRECTION('ref_axis',(1.,0.,0.));
#70581=DIRECTION('center_axis',(0.,0.,1.));
#70582=DIRECTION('ref_axis',(1.,0.,0.));
#70583=DIRECTION('',(0.,0.,-1.));
#70584=DIRECTION('center_axis',(0.,0.,-1.));
#70585=DIRECTION('ref_axis',(1.,0.,0.));
#70586=DIRECTION('center_axis',(0.,0.,1.));
#70587=DIRECTION('ref_axis',(1.,0.,0.));
#70588=DIRECTION('',(-0.707106781186547,-8.65956056235493E-17,-0.707106781186547));
#70589=DIRECTION('center_axis',(0.,0.,1.));
#70590=DIRECTION('ref_axis',(1.,0.,0.));
#70591=DIRECTION('center_axis',(0.,0.,1.));
#70592=DIRECTION('ref_axis',(1.,0.,0.));
#70593=DIRECTION('center_axis',(0.,0.,1.));
#70594=DIRECTION('ref_axis',(1.,0.,0.));
#70595=DIRECTION('center_axis',(0.,0.,1.));
#70596=DIRECTION('ref_axis',(1.,0.,0.));
#70597=DIRECTION('center_axis',(0.,0.,1.));
#70598=DIRECTION('ref_axis',(1.,0.,0.));
#70599=DIRECTION('center_axis',(0.,0.,1.));
#70600=DIRECTION('ref_axis',(1.,0.,0.));
#70601=DIRECTION('center_axis',(0.,0.,1.));
#70602=DIRECTION('ref_axis',(1.,0.,0.));
#70603=DIRECTION('center_axis',(0.,0.,1.));
#70604=DIRECTION('ref_axis',(1.,0.,0.));
#70605=DIRECTION('center_axis',(0.,0.,1.));
#70606=DIRECTION('ref_axis',(1.,0.,0.));
#70607=DIRECTION('center_axis',(0.,0.,1.));
#70608=DIRECTION('ref_axis',(1.,0.,0.));
#70609=DIRECTION('center_axis',(0.,0.,1.));
#70610=DIRECTION('ref_axis',(1.,0.,0.));
#70611=DIRECTION('center_axis',(0.,0.,1.));
#70612=DIRECTION('ref_axis',(1.,0.,0.));
#70613=DIRECTION('center_axis',(0.,0.,1.));
#70614=DIRECTION('ref_axis',(1.,0.,0.));
#70615=DIRECTION('center_axis',(0.,0.,1.));
#70616=DIRECTION('ref_axis',(1.,0.,0.));
#70617=DIRECTION('center_axis',(0.,0.,1.));
#70618=DIRECTION('ref_axis',(1.,0.,0.));
#70619=DIRECTION('center_axis',(0.,0.,1.));
#70620=DIRECTION('ref_axis',(1.,0.,0.));
#70621=DIRECTION('center_axis',(0.,0.,1.));
#70622=DIRECTION('ref_axis',(1.,0.,0.));
#70623=DIRECTION('center_axis',(0.,0.,1.));
#70624=DIRECTION('ref_axis',(1.,0.,0.));
#70625=DIRECTION('center_axis',(0.,0.,1.));
#70626=DIRECTION('ref_axis',(1.,0.,0.));
#70627=DIRECTION('center_axis',(0.,0.,1.));
#70628=DIRECTION('ref_axis',(1.,0.,0.));
#70629=DIRECTION('center_axis',(0.,0.,1.));
#70630=DIRECTION('ref_axis',(1.,0.,0.));
#70631=DIRECTION('center_axis',(0.,0.,1.));
#70632=DIRECTION('ref_axis',(1.,0.,0.));
#70633=DIRECTION('center_axis',(0.,0.,1.));
#70634=DIRECTION('ref_axis',(1.,0.,0.));
#70635=DIRECTION('center_axis',(0.,0.,1.));
#70636=DIRECTION('ref_axis',(1.,0.,0.));
#70637=DIRECTION('center_axis',(0.,0.,1.));
#70638=DIRECTION('ref_axis',(1.,0.,0.));
#70639=DIRECTION('center_axis',(0.,0.,1.));
#70640=DIRECTION('ref_axis',(1.,0.,0.));
#70641=DIRECTION('center_axis',(0.,0.,1.));
#70642=DIRECTION('ref_axis',(1.,0.,0.));
#70643=DIRECTION('center_axis',(0.,0.,1.));
#70644=DIRECTION('ref_axis',(1.,0.,0.));
#70645=DIRECTION('center_axis',(0.,0.,1.));
#70646=DIRECTION('ref_axis',(1.,0.,0.));
#70647=DIRECTION('center_axis',(0.,0.,1.));
#70648=DIRECTION('ref_axis',(1.,0.,0.));
#70649=DIRECTION('center_axis',(0.,0.,1.));
#70650=DIRECTION('ref_axis',(1.,0.,0.));
#70651=DIRECTION('center_axis',(0.,0.,1.));
#70652=DIRECTION('ref_axis',(1.,0.,0.));
#70653=DIRECTION('center_axis',(0.,0.,1.));
#70654=DIRECTION('ref_axis',(1.,0.,0.));
#70655=DIRECTION('center_axis',(0.,0.,1.));
#70656=DIRECTION('ref_axis',(1.,0.,0.));
#70657=DIRECTION('center_axis',(0.,0.,1.));
#70658=DIRECTION('ref_axis',(1.,0.,0.));
#70659=DIRECTION('center_axis',(0.,0.,1.));
#70660=DIRECTION('ref_axis',(1.,0.,0.));
#70661=DIRECTION('center_axis',(0.,0.,1.));
#70662=DIRECTION('ref_axis',(1.,0.,0.));
#70663=DIRECTION('center_axis',(-0.09993150545836,0.994994318685703,0.));
#70664=DIRECTION('ref_axis',(0.994994318685703,0.09993150545836,0.));
#70665=DIRECTION('',(0.,0.,-1.));
#70666=DIRECTION('center_axis',(-0.863705578271065,-0.503996700448967,0.));
#70667=DIRECTION('ref_axis',(-0.503996700448967,0.863705578271065,0.));
#70668=DIRECTION('',(0.,0.,1.));
#70669=DIRECTION('center_axis',(0.0569502211623254,0.998377019121315,0.));
#70670=DIRECTION('ref_axis',(0.998377019121315,-0.0569502211623254,0.));
#70671=DIRECTION('',(0.,0.,-1.));
#70672=DIRECTION('',(0.,0.,-1.));
#70673=DIRECTION('center_axis',(-0.931914383582088,-0.362678344642767,0.));
#70674=DIRECTION('ref_axis',(-0.362678344642767,0.931914383582087,0.));
#70675=DIRECTION('',(0.,0.,1.));
#70676=DIRECTION('center_axis',(0.,0.,1.));
#70677=DIRECTION('ref_axis',(1.,0.,0.));
#70678=DIRECTION('',(0.,0.,-1.));
#70679=DIRECTION('center_axis',(0.,0.,1.));
#70680=DIRECTION('ref_axis',(1.,0.,0.));
#70681=DIRECTION('center_axis',(-0.9771763639228,-0.212429644331046,0.));
#70682=DIRECTION('ref_axis',(-0.212429644331046,0.9771763639228,0.));
#70683=DIRECTION('',(0.,0.,-1.));
#70684=DIRECTION('',(0.,0.,1.));
#70685=DIRECTION('center_axis',(0.212429644331046,0.9771763639228,0.));
#70686=DIRECTION('ref_axis',(0.9771763639228,-0.212429644331046,0.));
#70687=DIRECTION('center_axis',(0.,0.,1.));
#70688=DIRECTION('ref_axis',(1.,0.,0.));
#70689=DIRECTION('',(0.,0.,-1.));
#70690=DIRECTION('center_axis',(0.362678344642768,0.931914383582087,0.));
#70691=DIRECTION('ref_axis',(0.931914383582087,-0.362678344642768,0.));
#70692=DIRECTION('',(0.,0.,-1.));
#70693=DIRECTION('center_axis',(-0.998377019121315,-0.0569502211623249,
0.));
#70694=DIRECTION('ref_axis',(-0.0569502211623248,0.998377019121315,0.));
#70695=DIRECTION('',(0.,0.,1.));
#70696=DIRECTION('center_axis',(0.503996700448967,0.863705578271065,0.));
#70697=DIRECTION('ref_axis',(0.863705578271065,-0.503996700448967,0.));
#70698=DIRECTION('',(0.,0.,-1.));
#70699=DIRECTION('',(0.,0.,-1.));
#70700=DIRECTION('center_axis',(-0.994994318685703,0.0999315054583604,0.));
#70701=DIRECTION('ref_axis',(0.0999315054583604,0.994994318685703,0.));
#70702=DIRECTION('',(0.,0.,1.));
#70703=DIRECTION('center_axis',(0.,0.,1.));
#70704=DIRECTION('ref_axis',(1.,0.,0.));
#70705=DIRECTION('',(0.,0.,-1.));
#70706=DIRECTION('center_axis',(0.,0.,1.));
#70707=DIRECTION('ref_axis',(1.,0.,0.));
#70708=DIRECTION('center_axis',(-0.967111555927228,0.254352586761009,0.));
#70709=DIRECTION('ref_axis',(0.254352586761009,0.967111555927228,0.));
#70710=DIRECTION('',(0.,0.,-1.));
#70711=DIRECTION('',(0.,0.,1.));
#70712=DIRECTION('center_axis',(0.632904984820962,0.774229475148536,0.));
#70713=DIRECTION('ref_axis',(0.774229475148536,-0.632904984820962,0.));
#70714=DIRECTION('center_axis',(0.,0.,1.));
#70715=DIRECTION('ref_axis',(1.,0.,0.));
#70716=DIRECTION('',(0.,0.,-1.));
#70717=DIRECTION('center_axis',(0.746229047975447,0.665689272827539,0.));
#70718=DIRECTION('ref_axis',(0.665689272827539,-0.746229047975447,0.));
#70719=DIRECTION('',(0.,0.,-1.));
#70720=DIRECTION('center_axis',(-0.915415297002588,0.402510663229763,0.));
#70721=DIRECTION('ref_axis',(0.402510663229763,0.915415297002588,0.));
#70722=DIRECTION('',(0.,0.,1.));
#70723=DIRECTION('center_axis',(0.841178475376555,0.540757591313496,0.));
#70724=DIRECTION('ref_axis',(0.540757591313496,-0.841178475376555,0.));
#70725=DIRECTION('',(0.,0.,-1.));
#70726=DIRECTION('',(0.,0.,-1.));
#70727=DIRECTION('center_axis',(-0.841178475376555,0.540757591313497,0.));
#70728=DIRECTION('ref_axis',(0.540757591313497,0.841178475376555,0.));
#70729=DIRECTION('',(0.,0.,1.));
#70730=DIRECTION('center_axis',(0.,0.,1.));
#70731=DIRECTION('ref_axis',(1.,0.,0.));
#70732=DIRECTION('',(0.,0.,-1.));
#70733=DIRECTION('center_axis',(0.,0.,1.));
#70734=DIRECTION('ref_axis',(1.,0.,0.));
#70735=DIRECTION('center_axis',(-0.746229047975447,0.66568927282754,0.));
#70736=DIRECTION('ref_axis',(0.66568927282754,0.746229047975447,0.));
#70737=DIRECTION('',(0.,0.,-1.));
#70738=DIRECTION('',(0.,0.,1.));
#70739=DIRECTION('center_axis',(0.915415297002588,0.402510663229763,0.));
#70740=DIRECTION('ref_axis',(0.402510663229763,-0.915415297002588,0.));
#70741=DIRECTION('center_axis',(0.,0.,1.));
#70742=DIRECTION('ref_axis',(1.,0.,0.));
#70743=DIRECTION('',(0.,0.,-1.));
#70744=DIRECTION('center_axis',(0.967111555927228,0.254352586761009,0.));
#70745=DIRECTION('ref_axis',(0.254352586761008,-0.967111555927228,0.));
#70746=DIRECTION('',(0.,0.,-1.));
#70747=DIRECTION('center_axis',(-0.632904984820962,0.774229475148536,0.));
#70748=DIRECTION('ref_axis',(0.774229475148536,0.632904984820962,0.));
#70749=DIRECTION('',(0.,0.,1.));
#70750=DIRECTION('center_axis',(0.994994318685703,0.0999315054583601,0.));
#70751=DIRECTION('ref_axis',(0.0999315054583601,-0.994994318685703,0.));
#70752=DIRECTION('',(0.,0.,-1.));
#70753=DIRECTION('',(0.,0.,-1.));
#70754=DIRECTION('center_axis',(-0.503996700448967,0.863705578271065,0.));
#70755=DIRECTION('ref_axis',(0.863705578271065,0.503996700448967,0.));
#70756=DIRECTION('',(0.,0.,1.));
#70757=DIRECTION('center_axis',(0.,0.,1.));
#70758=DIRECTION('ref_axis',(1.,0.,0.));
#70759=DIRECTION('',(0.,0.,-1.));
#70760=DIRECTION('center_axis',(0.,0.,1.));
#70761=DIRECTION('ref_axis',(1.,0.,0.));
#70762=DIRECTION('center_axis',(-0.362678344642767,0.931914383582087,0.));
#70763=DIRECTION('ref_axis',(0.931914383582087,0.362678344642767,0.));
#70764=DIRECTION('',(0.,0.,-1.));
#70765=DIRECTION('',(0.,0.,1.));
#70766=DIRECTION('center_axis',(0.998377019121315,-0.0569502211623253,0.));
#70767=DIRECTION('ref_axis',(-0.0569502211623253,-0.998377019121315,0.));
#70768=DIRECTION('center_axis',(0.,0.,1.));
#70769=DIRECTION('ref_axis',(1.,0.,0.));
#70770=DIRECTION('',(0.,0.,-1.));
#70771=DIRECTION('center_axis',(0.9771763639228,-0.212429644331046,0.));
#70772=DIRECTION('ref_axis',(-0.212429644331046,-0.9771763639228,0.));
#70773=DIRECTION('',(0.,0.,-1.));
#70774=DIRECTION('center_axis',(-0.212429644331046,0.9771763639228,0.));
#70775=DIRECTION('ref_axis',(0.9771763639228,0.212429644331046,0.));
#70776=DIRECTION('',(0.,0.,1.));
#70777=DIRECTION('center_axis',(0.931914383582087,-0.362678344642768,0.));
#70778=DIRECTION('ref_axis',(-0.362678344642768,-0.931914383582087,0.));
#70779=DIRECTION('',(0.,0.,-1.));
#70780=DIRECTION('',(0.,0.,-1.));
#70781=DIRECTION('center_axis',(-0.056950221162325,0.998377019121315,0.));
#70782=DIRECTION('ref_axis',(0.998377019121315,0.056950221162325,0.));
#70783=DIRECTION('',(0.,0.,1.));
#70784=DIRECTION('center_axis',(0.,0.,1.));
#70785=DIRECTION('ref_axis',(1.,0.,0.));
#70786=DIRECTION('',(0.,0.,-1.));
#70787=DIRECTION('center_axis',(0.,0.,1.));
#70788=DIRECTION('ref_axis',(1.,0.,0.));
#70789=DIRECTION('center_axis',(0.0999315054583604,0.994994318685703,0.));
#70790=DIRECTION('ref_axis',(0.994994318685703,-0.0999315054583604,0.));
#70791=DIRECTION('',(0.,0.,-1.));
#70792=DIRECTION('',(0.,0.,1.));
#70793=DIRECTION('center_axis',(0.863705578271065,-0.503996700448967,0.));
#70794=DIRECTION('ref_axis',(-0.503996700448967,-0.863705578271065,0.));
#70795=DIRECTION('center_axis',(0.,0.,1.));
#70796=DIRECTION('ref_axis',(1.,0.,0.));
#70797=DIRECTION('',(0.,0.,-1.));
#70798=DIRECTION('center_axis',(0.774229475148536,-0.632904984820962,0.));
#70799=DIRECTION('ref_axis',(-0.632904984820962,-0.774229475148536,0.));
#70800=DIRECTION('',(0.,0.,-1.));
#70801=DIRECTION('center_axis',(0.254352586761009,0.967111555927228,0.));
#70802=DIRECTION('ref_axis',(0.967111555927228,-0.254352586761009,0.));
#70803=DIRECTION('',(0.,0.,1.));
#70804=DIRECTION('center_axis',(0.665689272827539,-0.746229047975447,0.));
#70805=DIRECTION('ref_axis',(-0.746229047975447,-0.665689272827539,0.));
#70806=DIRECTION('',(0.,0.,-1.));
#70807=DIRECTION('',(0.,0.,-1.));
#70808=DIRECTION('center_axis',(0.402510663229763,0.915415297002588,0.));
#70809=DIRECTION('ref_axis',(0.915415297002588,-0.402510663229763,0.));
#70810=DIRECTION('',(0.,0.,1.));
#70811=DIRECTION('center_axis',(0.,0.,1.));
#70812=DIRECTION('ref_axis',(1.,0.,0.));
#70813=DIRECTION('',(0.,0.,-1.));
#70814=DIRECTION('center_axis',(0.,0.,1.));
#70815=DIRECTION('ref_axis',(1.,0.,0.));
#70816=DIRECTION('center_axis',(0.540757591313497,0.841178475376555,0.));
#70817=DIRECTION('ref_axis',(0.841178475376555,-0.540757591313497,0.));
#70818=DIRECTION('',(0.,0.,-1.));
#70819=DIRECTION('',(0.,0.,1.));
#70820=DIRECTION('center_axis',(0.540757591313496,-0.841178475376555,0.));
#70821=DIRECTION('ref_axis',(-0.841178475376555,-0.540757591313496,0.));
#70822=DIRECTION('center_axis',(0.,0.,1.));
#70823=DIRECTION('ref_axis',(1.,0.,0.));
#70824=DIRECTION('',(0.,0.,-1.));
#70825=DIRECTION('center_axis',(0.402510663229763,-0.915415297002588,0.));
#70826=DIRECTION('ref_axis',(-0.915415297002588,-0.402510663229763,0.));
#70827=DIRECTION('',(0.,0.,-1.));
#70828=DIRECTION('center_axis',(0.66568927282754,0.746229047975447,0.));
#70829=DIRECTION('ref_axis',(0.746229047975447,-0.66568927282754,0.));
#70830=DIRECTION('',(0.,0.,1.));
#70831=DIRECTION('center_axis',(0.254352586761009,-0.967111555927228,0.));
#70832=DIRECTION('ref_axis',(-0.967111555927228,-0.254352586761009,0.));
#70833=DIRECTION('',(0.,0.,-1.));
#70834=DIRECTION('',(0.,0.,-1.));
#70835=DIRECTION('center_axis',(0.774229475148536,0.632904984820962,0.));
#70836=DIRECTION('ref_axis',(0.632904984820962,-0.774229475148536,0.));
#70837=DIRECTION('',(0.,0.,1.));
#70838=DIRECTION('center_axis',(0.,0.,1.));
#70839=DIRECTION('ref_axis',(1.,0.,0.));
#70840=DIRECTION('',(0.,0.,-1.));
#70841=DIRECTION('center_axis',(0.,0.,1.));
#70842=DIRECTION('ref_axis',(1.,0.,0.));
#70843=DIRECTION('center_axis',(0.863705578271065,0.503996700448967,0.));
#70844=DIRECTION('ref_axis',(0.503996700448967,-0.863705578271065,0.));
#70845=DIRECTION('',(0.,0.,-1.));
#70846=DIRECTION('',(0.,0.,1.));
#70847=DIRECTION('center_axis',(0.0999315054583602,-0.994994318685703,0.));
#70848=DIRECTION('ref_axis',(-0.994994318685703,-0.0999315054583602,0.));
#70849=DIRECTION('center_axis',(0.,0.,1.));
#70850=DIRECTION('ref_axis',(1.,0.,0.));
#70851=DIRECTION('',(0.,0.,-1.));
#70852=DIRECTION('center_axis',(-0.0569502211623253,-0.998377019121315,
0.));
#70853=DIRECTION('ref_axis',(-0.998377019121315,0.0569502211623253,0.));
#70854=DIRECTION('',(0.,0.,-1.));
#70855=DIRECTION('center_axis',(0.931914383582087,0.362678344642767,0.));
#70856=DIRECTION('ref_axis',(0.362678344642767,-0.931914383582087,0.));
#70857=DIRECTION('',(0.,0.,1.));
#70858=DIRECTION('center_axis',(-0.212429644331046,-0.9771763639228,0.));
#70859=DIRECTION('ref_axis',(-0.9771763639228,0.212429644331046,0.));
#70860=DIRECTION('',(0.,0.,-1.));
#70861=DIRECTION('',(0.,0.,-1.));
#70862=DIRECTION('center_axis',(0.9771763639228,0.212429644331046,0.));
#70863=DIRECTION('ref_axis',(0.212429644331046,-0.9771763639228,0.));
#70864=DIRECTION('',(0.,0.,1.));
#70865=DIRECTION('center_axis',(0.,0.,1.));
#70866=DIRECTION('ref_axis',(1.,0.,0.));
#70867=DIRECTION('',(0.,0.,-1.));
#70868=DIRECTION('center_axis',(0.,0.,1.));
#70869=DIRECTION('ref_axis',(1.,0.,0.));
#70870=DIRECTION('center_axis',(0.998377019121315,0.056950221162325,0.));
#70871=DIRECTION('ref_axis',(0.056950221162325,-0.998377019121315,0.));
#70872=DIRECTION('',(0.,0.,-1.));
#70873=DIRECTION('',(0.,0.,1.));
#70874=DIRECTION('center_axis',(-0.362678344642768,-0.931914383582087,0.));
#70875=DIRECTION('ref_axis',(-0.931914383582087,0.362678344642768,0.));
#70876=DIRECTION('center_axis',(0.,0.,1.));
#70877=DIRECTION('ref_axis',(1.,0.,0.));
#70878=DIRECTION('',(0.,0.,-1.));
#70879=DIRECTION('center_axis',(-0.503996700448967,-0.863705578271065,0.));
#70880=DIRECTION('ref_axis',(-0.863705578271065,0.503996700448967,0.));
#70881=DIRECTION('',(0.,0.,-1.));
#70882=DIRECTION('center_axis',(0.994994318685703,-0.0999315054583603,0.));
#70883=DIRECTION('ref_axis',(-0.0999315054583603,-0.994994318685703,0.));
#70884=DIRECTION('',(0.,0.,1.));
#70885=DIRECTION('center_axis',(-0.632904984820962,-0.774229475148536,0.));
#70886=DIRECTION('ref_axis',(-0.774229475148536,0.632904984820962,0.));
#70887=DIRECTION('',(0.,0.,-1.));
#70888=DIRECTION('',(0.,0.,-1.));
#70889=DIRECTION('center_axis',(0.967111555927228,-0.254352586761009,0.));
#70890=DIRECTION('ref_axis',(-0.254352586761009,-0.967111555927228,0.));
#70891=DIRECTION('',(0.,0.,1.));
#70892=DIRECTION('center_axis',(0.,0.,1.));
#70893=DIRECTION('ref_axis',(1.,0.,0.));
#70894=DIRECTION('',(0.,0.,-1.));
#70895=DIRECTION('center_axis',(0.,0.,1.));
#70896=DIRECTION('ref_axis',(1.,0.,0.));
#70897=DIRECTION('center_axis',(0.915415297002588,-0.402510663229763,0.));
#70898=DIRECTION('ref_axis',(-0.402510663229763,-0.915415297002588,0.));
#70899=DIRECTION('',(0.,0.,-1.));
#70900=DIRECTION('',(0.,0.,1.));
#70901=DIRECTION('center_axis',(-0.746229047975447,-0.665689272827539,0.));
#70902=DIRECTION('ref_axis',(-0.665689272827539,0.746229047975447,0.));
#70903=DIRECTION('center_axis',(0.,0.,1.));
#70904=DIRECTION('ref_axis',(1.,0.,0.));
#70905=DIRECTION('',(0.,0.,-1.));
#70906=DIRECTION('center_axis',(-0.841178475376555,-0.540757591313497,0.));
#70907=DIRECTION('ref_axis',(-0.540757591313497,0.841178475376555,0.));
#70908=DIRECTION('',(0.,0.,-1.));
#70909=DIRECTION('center_axis',(0.841178475376555,-0.540757591313497,0.));
#70910=DIRECTION('ref_axis',(-0.540757591313497,-0.841178475376555,0.));
#70911=DIRECTION('',(0.,0.,1.));
#70912=DIRECTION('center_axis',(-0.915415297002588,-0.402510663229763,0.));
#70913=DIRECTION('ref_axis',(-0.402510663229763,0.915415297002588,0.));
#70914=DIRECTION('',(0.,0.,-1.));
#70915=DIRECTION('',(0.,0.,-1.));
#70916=DIRECTION('center_axis',(0.746229047975447,-0.66568927282754,0.));
#70917=DIRECTION('ref_axis',(-0.66568927282754,-0.746229047975447,0.));
#70918=DIRECTION('',(0.,0.,1.));
#70919=DIRECTION('center_axis',(0.,0.,1.));
#70920=DIRECTION('ref_axis',(1.,0.,0.));
#70921=DIRECTION('',(0.,0.,-1.));
#70922=DIRECTION('center_axis',(0.,0.,1.));
#70923=DIRECTION('ref_axis',(1.,0.,0.));
#70924=DIRECTION('center_axis',(0.632904984820962,-0.774229475148536,0.));
#70925=DIRECTION('ref_axis',(-0.774229475148536,-0.632904984820962,0.));
#70926=DIRECTION('',(0.,0.,-1.));
#70927=DIRECTION('',(0.,0.,1.));
#70928=DIRECTION('center_axis',(-0.967111555927228,-0.254352586761009,0.));
#70929=DIRECTION('ref_axis',(-0.254352586761009,0.967111555927228,0.));
#70930=DIRECTION('center_axis',(0.,0.,1.));
#70931=DIRECTION('ref_axis',(1.,0.,0.));
#70932=DIRECTION('',(0.,0.,-1.));
#70933=DIRECTION('center_axis',(-0.994994318685703,-0.0999315054583602,
0.));
#70934=DIRECTION('ref_axis',(-0.0999315054583602,0.994994318685703,0.));
#70935=DIRECTION('',(0.,0.,-1.));
#70936=DIRECTION('center_axis',(0.503996700448967,-0.863705578271065,0.));
#70937=DIRECTION('ref_axis',(-0.863705578271065,-0.503996700448967,0.));
#70938=DIRECTION('',(0.,0.,1.));
#70939=DIRECTION('center_axis',(-0.998377019121315,0.0569502211623251,0.));
#70940=DIRECTION('ref_axis',(0.0569502211623251,0.998377019121315,0.));
#70941=DIRECTION('',(0.,0.,-1.));
#70942=DIRECTION('',(0.,0.,-1.));
#70943=DIRECTION('center_axis',(0.362678344642768,-0.931914383582087,0.));
#70944=DIRECTION('ref_axis',(-0.931914383582087,-0.362678344642768,0.));
#70945=DIRECTION('',(0.,0.,1.));
#70946=DIRECTION('center_axis',(0.,0.,1.));
#70947=DIRECTION('ref_axis',(1.,0.,0.));
#70948=DIRECTION('',(0.,0.,-1.));
#70949=DIRECTION('center_axis',(0.,0.,1.));
#70950=DIRECTION('ref_axis',(1.,0.,0.));
#70951=DIRECTION('center_axis',(0.212429644331046,-0.9771763639228,0.));
#70952=DIRECTION('ref_axis',(-0.9771763639228,-0.212429644331046,0.));
#70953=DIRECTION('',(0.,0.,-1.));
#70954=DIRECTION('',(0.,0.,1.));
#70955=DIRECTION('center_axis',(-0.9771763639228,0.212429644331046,0.));
#70956=DIRECTION('ref_axis',(0.212429644331046,0.9771763639228,0.));
#70957=DIRECTION('center_axis',(0.,0.,1.));
#70958=DIRECTION('ref_axis',(1.,0.,0.));
#70959=DIRECTION('',(0.,0.,-1.));
#70960=DIRECTION('center_axis',(-0.931914383582087,0.362678344642768,0.));
#70961=DIRECTION('ref_axis',(0.362678344642768,0.931914383582087,0.));
#70962=DIRECTION('',(0.,0.,-1.));
#70963=DIRECTION('center_axis',(0.0569502211623251,-0.998377019121315,0.));
#70964=DIRECTION('ref_axis',(-0.998377019121315,-0.0569502211623251,0.));
#70965=DIRECTION('',(0.,0.,1.));
#70966=DIRECTION('center_axis',(-0.863705578271065,0.503996700448967,0.));
#70967=DIRECTION('ref_axis',(0.503996700448967,0.863705578271065,0.));
#70968=DIRECTION('',(0.,0.,-1.));
#70969=DIRECTION('',(0.,0.,-1.));
#70970=DIRECTION('center_axis',(-0.0999315054583603,-0.994994318685703,
0.));
#70971=DIRECTION('ref_axis',(-0.994994318685703,0.0999315054583603,0.));
#70972=DIRECTION('',(0.,0.,1.));
#70973=DIRECTION('center_axis',(0.,0.,1.));
#70974=DIRECTION('ref_axis',(1.,0.,0.));
#70975=DIRECTION('',(0.,0.,-1.));
#70976=DIRECTION('center_axis',(0.,0.,1.));
#70977=DIRECTION('ref_axis',(1.,0.,0.));
#70978=DIRECTION('center_axis',(-0.254352586761009,-0.967111555927228,0.));
#70979=DIRECTION('ref_axis',(-0.967111555927228,0.254352586761009,0.));
#70980=DIRECTION('',(0.,0.,-1.));
#70981=DIRECTION('',(0.,0.,1.));
#70982=DIRECTION('center_axis',(-0.774229475148536,0.632904984820962,0.));
#70983=DIRECTION('ref_axis',(0.632904984820962,0.774229475148536,0.));
#70984=DIRECTION('center_axis',(0.,0.,1.));
#70985=DIRECTION('ref_axis',(1.,0.,0.));
#70986=DIRECTION('',(0.,0.,-1.));
#70987=DIRECTION('center_axis',(-0.665689272827539,0.746229047975447,0.));
#70988=DIRECTION('ref_axis',(0.746229047975447,0.665689272827539,0.));
#70989=DIRECTION('',(0.,0.,-1.));
#70990=DIRECTION('center_axis',(-0.402510663229763,-0.915415297002588,0.));
#70991=DIRECTION('ref_axis',(-0.915415297002588,0.402510663229763,0.));
#70992=DIRECTION('',(0.,0.,1.));
#70993=DIRECTION('center_axis',(-0.540757591313497,0.841178475376555,0.));
#70994=DIRECTION('ref_axis',(0.841178475376555,0.540757591313497,0.));
#70995=DIRECTION('',(0.,0.,-1.));
#70996=DIRECTION('',(0.,0.,-1.));
#70997=DIRECTION('center_axis',(-0.540757591313497,-0.841178475376555,0.));
#70998=DIRECTION('ref_axis',(-0.841178475376555,0.540757591313497,0.));
#70999=DIRECTION('center_axis',(0.,0.,-1.));
#71000=DIRECTION('ref_axis',(1.,0.,0.));
#71001=DIRECTION('center_axis',(0.,0.,1.));
#71002=DIRECTION('ref_axis',(1.,0.,0.));
#71003=DIRECTION('',(-0.707106781186547,-8.65956056235493E-17,-0.707106781186547));
#71004=DIRECTION('center_axis',(0.,0.,1.));
#71005=DIRECTION('ref_axis',(1.,0.,0.));
#71006=DIRECTION('center_axis',(0.,0.,-1.));
#71007=DIRECTION('ref_axis',(-1.,0.,0.));
#71008=DIRECTION('center_axis',(0.,0.,1.));
#71009=DIRECTION('ref_axis',(1.,0.,0.));
#71010=DIRECTION('center_axis',(0.,0.,1.));
#71011=DIRECTION('ref_axis',(1.,0.,0.));
#71012=DIRECTION('center_axis',(0.,0.,1.));
#71013=DIRECTION('ref_axis',(1.,0.,0.));
#71014=DIRECTION('',(0.707106781186548,8.65956056235493E-17,-0.707106781186548));
#71015=DIRECTION('center_axis',(0.,0.,1.));
#71016=DIRECTION('ref_axis',(1.,0.,0.));
#71017=DIRECTION('center_axis',(0.,0.,1.));
#71018=DIRECTION('ref_axis',(1.,0.,0.));
#71019=DIRECTION('',(0.,0.,-1.));
#71020=DIRECTION('center_axis',(0.,0.,1.));
#71021=DIRECTION('ref_axis',(1.,0.,0.));
#71022=DIRECTION('center_axis',(0.,0.,1.));
#71023=DIRECTION('ref_axis',(1.,0.,0.));
#71024=DIRECTION('',(0.707106781186555,8.65956056235503E-17,-0.70710678118654));
#71025=DIRECTION('center_axis',(0.,0.,-1.));
#71026=DIRECTION('ref_axis',(-1.,0.,0.));
#71027=DIRECTION('center_axis',(0.,0.,1.));
#71028=DIRECTION('ref_axis',(1.,0.,0.));
#71029=DIRECTION('center_axis',(0.,0.,1.));
#71030=DIRECTION('ref_axis',(1.,0.,0.));
#71031=DIRECTION('center_axis',(0.,0.,1.));
#71032=DIRECTION('ref_axis',(1.,0.,0.));
#71033=DIRECTION('',(0.,0.,-1.));
#71034=DIRECTION('center_axis',(0.,0.,1.));
#71035=DIRECTION('ref_axis',(1.,0.,0.));
#71036=DIRECTION('center_axis',(0.,0.,1.));
#71037=DIRECTION('ref_axis',(1.,0.,0.));
#71038=DIRECTION('',(0.707106781186555,8.65956056235503E-17,-0.70710678118654));
#71039=DIRECTION('center_axis',(0.,0.,-1.));
#71040=DIRECTION('ref_axis',(-1.,0.,0.));
#71041=DIRECTION('center_axis',(0.,0.,1.));
#71042=DIRECTION('ref_axis',(1.,0.,0.));
#71043=DIRECTION('center_axis',(0.,0.,1.));
#71044=DIRECTION('ref_axis',(1.,0.,0.));
#71045=DIRECTION('center_axis',(0.,0.,1.));
#71046=DIRECTION('ref_axis',(1.,0.,0.));
#71047=DIRECTION('center_axis',(0.,0.,1.));
#71048=DIRECTION('ref_axis',(1.,0.,0.));
#71049=DIRECTION('',(0.707106781186547,8.65956056235494E-17,-0.707106781186547));
#71050=DIRECTION('center_axis',(0.,0.,1.));
#71051=DIRECTION('ref_axis',(1.,0.,0.));
#71052=DIRECTION('center_axis',(0.,0.,1.));
#71053=DIRECTION('ref_axis',(1.,0.,0.));
#71054=DIRECTION('center_axis',(0.,0.,-1.));
#71055=DIRECTION('ref_axis',(1.,0.,0.));
#71056=DIRECTION('',(-0.8583968680612,-1.05123297686926E-16,-0.512986176132187));
#71057=DIRECTION('center_axis',(0.,0.,1.));
#71058=DIRECTION('ref_axis',(1.,0.,0.));
#71059=DIRECTION('center_axis',(0.,0.,1.));
#71060=DIRECTION('ref_axis',(1.,0.,0.));
#71061=DIRECTION('',(0.,0.,-1.));
#97718=CARTESIAN_POINT('',(0.,0.,0.));
#97719=CARTESIAN_POINT('Origin',(110.,20.,63.));
#97720=CARTESIAN_POINT('',(108.483391942524,20.,62.6800000000001));
#97721=CARTESIAN_POINT('',(108.483391942524,20.,63.3199999999999));
#97722=CARTESIAN_POINT('',(108.483391942524,20.,64.05));
#97723=CARTESIAN_POINT('',(108.45,20.,63.));
#97724=CARTESIAN_POINT('Origin',(110.,20.,63.));
#97725=CARTESIAN_POINT('Origin',(110.,20.,63.));
#97726=CARTESIAN_POINT('Origin',(110.,24.,63.));
#97727=CARTESIAN_POINT('',(110.,24.,64.55));
#97728=CARTESIAN_POINT('',(108.45,23.7963350489771,63.));
#97729=CARTESIAN_POINT('Ctrl Pts',(110.,24.,64.55));
#97730=CARTESIAN_POINT('Ctrl Pts',(109.804434914878,24.,64.55));
#97731=CARTESIAN_POINT('Ctrl Pts',(109.596431057671,23.9894828311411,64.5107353587906));
#97732=CARTESIAN_POINT('Ctrl Pts',(109.214794582034,23.9514893035012,64.3522727655961));
#97733=CARTESIAN_POINT('Ctrl Pts',(109.041091716494,23.9245204206378,64.233122738172));
#97734=CARTESIAN_POINT('Ctrl Pts',(108.766855310829,23.8735685672227,63.9588863325073));
#97735=CARTESIAN_POINT('Ctrl Pts',(108.647722381438,23.8461953948893,63.7851925753203));
#97736=CARTESIAN_POINT('Ctrl Pts',(108.489272290211,23.8072676307453,63.4035885188397));
#97737=CARTESIAN_POINT('Ctrl Pts',(108.45,23.7963350489771,63.19559639528));
#97738=CARTESIAN_POINT('Ctrl Pts',(108.45,23.7963350489771,63.));
#97739=CARTESIAN_POINT('',(110.,24.,61.45));
#97740=CARTESIAN_POINT('Ctrl Pts',(110.,24.,61.45));
#97741=CARTESIAN_POINT('Ctrl Pts',(110.195565085122,24.,61.45));
#97742=CARTESIAN_POINT('Ctrl Pts',(110.403568942329,23.9894828311411,61.4892646412094));
#97743=CARTESIAN_POINT('Ctrl Pts',(110.785205417966,23.9514893035012,61.6477272344039));
#97744=CARTESIAN_POINT('Ctrl Pts',(110.958908283506,23.9245204206378,61.766877261828));
#97745=CARTESIAN_POINT('Ctrl Pts',(111.233144689171,23.8735685672227,62.0411136674927));
#97746=CARTESIAN_POINT('Ctrl Pts',(111.352277618562,23.8461953948893,62.2148074246797));
#97747=CARTESIAN_POINT('Ctrl Pts',(111.510727709789,23.8072676307453,62.5964114811603));
#97748=CARTESIAN_POINT('Ctrl Pts',(111.55,23.7963350489771,62.80440360472));
#97749=CARTESIAN_POINT('Ctrl Pts',(111.55,23.7963350489771,63.));
#97750=CARTESIAN_POINT('Ctrl Pts',(111.55,23.7963350489771,63.19559639528));
#97751=CARTESIAN_POINT('Ctrl Pts',(111.510727709789,23.8072676307453,63.4035885188397));
#97752=CARTESIAN_POINT('Ctrl Pts',(111.352277618562,23.8461953948893,63.7851925753203));
#97753=CARTESIAN_POINT('Ctrl Pts',(111.233144689171,23.8735685672227,63.9588863325073));
#97754=CARTESIAN_POINT('Ctrl Pts',(110.958908283506,23.9245204206378,64.233122738172));
#97755=CARTESIAN_POINT('Ctrl Pts',(110.785205417966,23.9514893035012,64.3522727655961));
#97756=CARTESIAN_POINT('Ctrl Pts',(110.403568942329,23.9894828311411,64.5107353587906));
#97757=CARTESIAN_POINT('Ctrl Pts',(110.195565085122,24.,64.55));
#97758=CARTESIAN_POINT('Ctrl Pts',(110.,24.,64.55));
#97759=CARTESIAN_POINT('Ctrl Pts',(108.45,23.7963350489771,63.));
#97760=CARTESIAN_POINT('Ctrl Pts',(108.45,23.7963350489771,62.80440360472));
#97761=CARTESIAN_POINT('Ctrl Pts',(108.489272290211,23.8072676307453,62.5964114811603));
#97762=CARTESIAN_POINT('Ctrl Pts',(108.647722381438,23.8461953948893,62.2148074246797));
#97763=CARTESIAN_POINT('Ctrl Pts',(108.766855310829,23.8735685672227,62.0411136674927));
#97764=CARTESIAN_POINT('Ctrl Pts',(109.041091716494,23.9245204206378,61.766877261828));
#97765=CARTESIAN_POINT('Ctrl Pts',(109.214794582034,23.9514893035012,61.6477272344039));
#97766=CARTESIAN_POINT('Ctrl Pts',(109.596431057671,23.9894828311411,61.4892646412094));
#97767=CARTESIAN_POINT('Ctrl Pts',(109.804434914878,24.,61.45));
#97768=CARTESIAN_POINT('Ctrl Pts',(110.,24.,61.45));
#97769=CARTESIAN_POINT('',(108.45,24.,63.));
#97770=CARTESIAN_POINT('',(111.516608057476,20.,62.6800000000001));
#97771=CARTESIAN_POINT('Ctrl Pts',(111.516608057476,20.,62.6800000000001));
#97772=CARTESIAN_POINT('Ctrl Pts',(111.496300804331,20.0153990718724,62.5837558007975));
#97773=CARTESIAN_POINT('Ctrl Pts',(111.466684099523,20.0374168042622,62.4892051739527));
#97774=CARTESIAN_POINT('Ctrl Pts',(111.34901672214,20.118881048826,62.2094698392625));
#97775=CARTESIAN_POINT('Ctrl Pts',(111.231113753811,20.1924895398432,62.0390827321322));
#97776=CARTESIAN_POINT('Ctrl Pts',(110.961922515843,20.3231491933349,61.7698914941652));
#97777=CARTESIAN_POINT('Ctrl Pts',(110.791272112782,20.3900618513488,61.6512969408763));
#97778=CARTESIAN_POINT('Ctrl Pts',(110.410718369409,20.4839117719612,61.4912183468773));
#97779=CARTESIAN_POINT('Ctrl Pts',(110.200494469465,20.51,61.45));
#97780=CARTESIAN_POINT('Ctrl Pts',(109.799505530535,20.51,61.45));
#97781=CARTESIAN_POINT('Ctrl Pts',(109.589281630591,20.4839117719612,61.4912183468773));
#97782=CARTESIAN_POINT('Ctrl Pts',(109.208727887218,20.3900618513488,61.6512969408763));
#97783=CARTESIAN_POINT('Ctrl Pts',(109.038077484157,20.3231491933349,61.7698914941652));
#97784=CARTESIAN_POINT('Ctrl Pts',(108.768886246189,20.1924895398432,62.0390827321322));
#97785=CARTESIAN_POINT('Ctrl Pts',(108.65098327786,20.118881048826,62.2094698392625));
#97786=CARTESIAN_POINT('Ctrl Pts',(108.533315900477,20.0374168042622,62.4892051739528));
#97787=CARTESIAN_POINT('Ctrl Pts',(108.503699195669,20.0153990718724,62.5837558007975));
#97788=CARTESIAN_POINT('Ctrl Pts',(108.483391942524,20.,62.6800000000001));
#97789=CARTESIAN_POINT('',(111.516608057476,20.,63.3199999999999));
#97790=CARTESIAN_POINT('Origin',(110.,20.,63.));
#97791=CARTESIAN_POINT('Ctrl Pts',(108.483391942524,20.,63.3199999999999));
#97792=CARTESIAN_POINT('Ctrl Pts',(108.503699195669,20.0153990718724,63.4162441992025));
#97793=CARTESIAN_POINT('Ctrl Pts',(108.533315900477,20.0374168042622,63.5107948260473));
#97794=CARTESIAN_POINT('Ctrl Pts',(108.65098327786,20.118881048826,63.7905301607375));
#97795=CARTESIAN_POINT('Ctrl Pts',(108.768886246189,20.1924895398432,63.9609172678678));
#97796=CARTESIAN_POINT('Ctrl Pts',(109.038077484157,20.3231491933349,64.2301085058348));
#97797=CARTESIAN_POINT('Ctrl Pts',(109.208727887218,20.3900618513488,64.3487030591237));
#97798=CARTESIAN_POINT('Ctrl Pts',(109.589281630591,20.4839117719612,64.5087816531227));
#97799=CARTESIAN_POINT('Ctrl Pts',(109.799505530535,20.51,64.55));
#97800=CARTESIAN_POINT('Ctrl Pts',(110.200494469465,20.51,64.55));
#97801=CARTESIAN_POINT('Ctrl Pts',(110.410718369409,20.4839117719612,64.5087816531227));
#97802=CARTESIAN_POINT('Ctrl Pts',(110.791272112782,20.3900618513488,64.3487030591237));
#97803=CARTESIAN_POINT('Ctrl Pts',(110.961922515843,20.3231491933349,64.2301085058348));
#97804=CARTESIAN_POINT('Ctrl Pts',(111.231113753811,20.1924895398432,63.9609172678678));
#97805=CARTESIAN_POINT('Ctrl Pts',(111.34901672214,20.118881048826,63.7905301607375));
#97806=CARTESIAN_POINT('Ctrl Pts',(111.466684099523,20.0374168042622,63.5107948260473));
#97807=CARTESIAN_POINT('Ctrl Pts',(111.496300804331,20.0153990718724,63.4162441992025));
#97808=CARTESIAN_POINT('Ctrl Pts',(111.516608057476,20.,63.3199999999999));
#97809=CARTESIAN_POINT('Origin',(110.,20.,63.));
#97810=CARTESIAN_POINT('',(111.516608057476,20.,64.05));
#97811=CARTESIAN_POINT('Origin',(119.481808069713,16.4982291356138,81.));
#97812=CARTESIAN_POINT('',(119.481808069713,16.4982291356138,80.6));
#97813=CARTESIAN_POINT('',(119.913569220132,16.6880757195422,80.2));
#97814=CARTESIAN_POINT('Ctrl Pts',(119.481808069713,16.4982291356138,80.6));
#97815=CARTESIAN_POINT('Ctrl Pts',(119.693282918898,16.5912152175378,80.4056749851136));
#97816=CARTESIAN_POINT('Ctrl Pts',(119.913569220132,16.6880757195422,80.2));
#97817=CARTESIAN_POINT('',(119.481808069713,16.4982291356138,66.4));
#97818=CARTESIAN_POINT('',(119.481808069713,16.4982291356138,81.));
#97819=CARTESIAN_POINT('',(119.913569220132,16.6880757195422,66.8));
#97820=CARTESIAN_POINT('Ctrl Pts',(119.913569220132,16.6880757195423,66.8));
#97821=CARTESIAN_POINT('Ctrl Pts',(119.693282918896,16.5912152175369,66.5943250148847));
#97822=CARTESIAN_POINT('Ctrl Pts',(119.481808069713,16.4982291356138,66.4));
#97823=CARTESIAN_POINT('',(119.913569220132,16.6880757195422,73.5));
#97824=CARTESIAN_POINT('Origin',(120.102794398862,15.9442652568178,81.));
#97825=CARTESIAN_POINT('',(119.833771504544,16.184252771882,80.2));
#97826=CARTESIAN_POINT('Ctrl Pts',(119.833771504544,16.184252771882,80.2));
#97827=CARTESIAN_POINT('Ctrl Pts',(119.654198323508,16.3444447941938,80.4056749851128));
#97828=CARTESIAN_POINT('Ctrl Pts',(119.481808069713,16.4982291356138,80.6));
#97829=CARTESIAN_POINT('',(119.833771504544,16.184252771882,66.8));
#97830=CARTESIAN_POINT('',(119.833771504544,16.184252771882,73.5));
#97831=CARTESIAN_POINT('Ctrl Pts',(119.481808069713,16.4982291356138,66.4));
#97832=CARTESIAN_POINT('Ctrl Pts',(119.654198323507,16.344444794195,66.5943250148856));
#97833=CARTESIAN_POINT('Ctrl Pts',(119.833771504544,16.184252771882,66.8));
#97834=CARTESIAN_POINT('Origin',(110.,18.,66.4));
#97835=CARTESIAN_POINT('',(119.58628655942,15.1534037868576,66.8));
#97836=CARTESIAN_POINT('Origin',(110.,18.,66.8));
#97837=CARTESIAN_POINT('',(119.130142556433,15.0334368540005,66.4));
#97838=CARTESIAN_POINT('Ctrl Pts',(119.58628655942,15.1534037868576,66.8));
#97839=CARTESIAN_POINT('Ctrl Pts',(119.353560027287,15.0921961680536,66.5943250148888));
#97840=CARTESIAN_POINT('Ctrl Pts',(119.130142556433,15.0334368540005,66.4));
#97841=CARTESIAN_POINT('',(119.428656012836,14.6682668486787,66.8));
#97842=CARTESIAN_POINT('Ctrl Pts',(119.130142556433,15.0334368540005,66.4));
#97843=CARTESIAN_POINT('Ctrl Pts',(119.276353228958,14.8545780758826,66.5943250148879));
#97844=CARTESIAN_POINT('Ctrl Pts',(119.428656012836,14.6682668486787,66.8));
#97845=CARTESIAN_POINT('',(119.022957708555,13.6888245002517,66.8));
#97846=CARTESIAN_POINT('Origin',(110.,18.,66.8));
#97847=CARTESIAN_POINT('',(118.553662632208,13.6416912025004,66.4));
#97848=CARTESIAN_POINT('Ctrl Pts',(119.022957708555,13.6888245002517,66.8));
#97849=CARTESIAN_POINT('Ctrl Pts',(118.783521445114,13.6647768993582,66.5943250148874));
#97850=CARTESIAN_POINT('Ctrl Pts',(118.553662632208,13.6416912025004,66.4));
#97851=CARTESIAN_POINT('',(118.791375718177,13.2343192530493,66.8));
#97852=CARTESIAN_POINT('Ctrl Pts',(118.553662632208,13.6416912025004,66.4));
#97853=CARTESIAN_POINT('Ctrl Pts',(118.670093531459,13.4421620844006,66.594325014888));
#97854=CARTESIAN_POINT('Ctrl Pts',(118.791375718177,13.2343192530493,66.8));
#97855=CARTESIAN_POINT('',(118.237453693425,12.3304006624208,66.8));
#97856=CARTESIAN_POINT('Origin',(110.,18.,66.8));
#97857=CARTESIAN_POINT('',(117.766563145999,12.3572615779923,66.4));
#97858=CARTESIAN_POINT('Ctrl Pts',(118.237453693425,12.3304006624208,66.8));
#97859=CARTESIAN_POINT('Ctrl Pts',(117.997203414127,12.3441052111817,66.5943250148877));
#97860=CARTESIAN_POINT('Ctrl Pts',(117.766563145999,12.3572615779923,66.4));
#97861=CARTESIAN_POINT('',(117.937622576432,11.9177185337975,66.8));
#97862=CARTESIAN_POINT('Ctrl Pts',(117.766563145999,12.3572615779923,66.4));
#97863=CARTESIAN_POINT('Ctrl Pts',(117.850347356823,12.1419751889999,66.5943250148858));
#97864=CARTESIAN_POINT('Ctrl Pts',(117.937622576432,11.9177185337974,66.8));
#97865=CARTESIAN_POINT('',(117.249116229822,11.1115811766025,66.8));
#97866=CARTESIAN_POINT('Origin',(110.,18.,66.8));
#97867=CARTESIAN_POINT('',(116.788225099391,11.2117749006091,66.4));
#97868=CARTESIAN_POINT('Ctrl Pts',(117.249116229822,11.1115811766024,66.8));
#97869=CARTESIAN_POINT('Ctrl Pts',(117.01396769389,11.1627004235442,66.5943250148884));
#97870=CARTESIAN_POINT('Ctrl Pts',(116.788225099391,11.2117749006091,66.4));
#97871=CARTESIAN_POINT('',(116.888418823398,10.7508837701784,66.8));
#97872=CARTESIAN_POINT('Ctrl Pts',(116.788225099391,11.2117749006091,66.4));
#97873=CARTESIAN_POINT('Ctrl Pts',(116.837299576456,10.9860323061102,66.5943250148886));
#97874=CARTESIAN_POINT('Ctrl Pts',(116.888418823398,10.7508837701784,66.8));
#97875=CARTESIAN_POINT('',(116.082281466203,10.0623774235676,66.8));
#97876=CARTESIAN_POINT('Origin',(110.,18.,66.8));
#97877=CARTESIAN_POINT('',(115.642738422008,10.2334368540005,66.4));
#97878=CARTESIAN_POINT('Ctrl Pts',(116.082281466203,10.0623774235676,66.8));
#97879=CARTESIAN_POINT('Ctrl Pts',(115.858024811002,10.1496526431758,66.5943250148877));
#97880=CARTESIAN_POINT('Ctrl Pts',(115.642738422008,10.2334368540005,66.4));
#97881=CARTESIAN_POINT('',(115.669599337579,9.762546306575,66.8));
#97882=CARTESIAN_POINT('Ctrl Pts',(115.642738422008,10.2334368540005,66.4));
#97883=CARTESIAN_POINT('Ctrl Pts',(115.655894788818,10.0027965858723,66.5943250148879));
#97884=CARTESIAN_POINT('Ctrl Pts',(115.669599337579,9.76254630657496,66.8));
#97885=CARTESIAN_POINT('',(114.765680746951,9.20862428182348,66.8));
#97886=CARTESIAN_POINT('Origin',(110.,18.,66.8));
#97887=CARTESIAN_POINT('',(114.3583087975,9.44633736779169,66.4));
#97888=CARTESIAN_POINT('Ctrl Pts',(114.765680746951,9.20862428182346,66.8));
#97889=CARTESIAN_POINT('Ctrl Pts',(114.557837915599,9.32990646854147,66.5943250148875));
#97890=CARTESIAN_POINT('Ctrl Pts',(114.3583087975,9.44633736779169,66.4));
#97891=CARTESIAN_POINT('',(114.311175499748,8.97704229144512,66.8));
#97892=CARTESIAN_POINT('Ctrl Pts',(114.3583087975,9.44633736779169,66.4));
#97893=CARTESIAN_POINT('Ctrl Pts',(114.335223100642,9.21647855488602,66.5943250148877));
#97894=CARTESIAN_POINT('Ctrl Pts',(114.311175499748,8.97704229144508,66.8));
#97895=CARTESIAN_POINT('',(113.331733151321,8.57134398716408,66.8));
#97896=CARTESIAN_POINT('Origin',(110.,18.,66.8));
#97897=CARTESIAN_POINT('',(112.966563146,8.86985744356654,66.4));
#97898=CARTESIAN_POINT('Ctrl Pts',(113.331733151321,8.57134398716406,66.8));
#97899=CARTESIAN_POINT('Ctrl Pts',(113.145421924117,8.72364677104231,66.5943250148875));
#97900=CARTESIAN_POINT('Ctrl Pts',(112.966563146,8.86985744356654,66.4));
#97901=CARTESIAN_POINT('',(112.846596213142,8.41371344057965,66.8));
#97902=CARTESIAN_POINT('Ctrl Pts',(112.966563146,8.86985744356654,66.4));
#97903=CARTESIAN_POINT('Ctrl Pts',(112.907803831947,8.64643997271467,66.5943250148877));
#97904=CARTESIAN_POINT('Ctrl Pts',(112.846596213142,8.41371344057961,66.8));
#97905=CARTESIAN_POINT('',(111.815747228118,8.16622849545598,66.8));
#97906=CARTESIAN_POINT('Origin',(110.,18.,66.8));
#97907=CARTESIAN_POINT('',(111.501770864386,8.51819193028669,66.4));
#97908=CARTESIAN_POINT('Ctrl Pts',(111.815747228118,8.16622849545595,66.8));
#97909=CARTESIAN_POINT('Ctrl Pts',(111.655555205807,8.34580167649132,66.5943250148875));
#97910=CARTESIAN_POINT('Ctrl Pts',(111.501770864386,8.51819193028669,66.4));
#97911=CARTESIAN_POINT('',(111.311924280458,8.08643077986816,66.8));
#97912=CARTESIAN_POINT('Ctrl Pts',(111.501770864386,8.51819193028669,66.4));
#97913=CARTESIAN_POINT('Ctrl Pts',(111.408784782462,8.3067170811009,66.5943250148878));
#97914=CARTESIAN_POINT('Ctrl Pts',(111.311924280458,8.08643077986812,66.8));
#97915=CARTESIAN_POINT('',(110.255051582039,8.00325309460625,66.8));
#97916=CARTESIAN_POINT('Origin',(110.,18.,66.8));
#97917=CARTESIAN_POINT('',(110.,8.40000000000002,66.4));
#97918=CARTESIAN_POINT('Ctrl Pts',(110.255051582039,8.00325309460621,66.8));
#97919=CARTESIAN_POINT('Ctrl Pts',(110.124923223856,8.20567498511282,66.5943250148871));
#97920=CARTESIAN_POINT('Ctrl Pts',(110.,8.40000000000002,66.4));
#97921=CARTESIAN_POINT('',(109.744948417961,8.00325309460625,66.8));
#97922=CARTESIAN_POINT('Ctrl Pts',(110.,8.40000000000002,66.4));
#97923=CARTESIAN_POINT('Ctrl Pts',(109.875076776144,8.20567498511234,66.5943250148876));
#97924=CARTESIAN_POINT('Ctrl Pts',(109.744948417961,8.00325309460622,66.8));
#97925=CARTESIAN_POINT('',(108.688075719542,8.08643077986816,66.8));
#97926=CARTESIAN_POINT('Origin',(110.,18.,66.8));
#97927=CARTESIAN_POINT('',(108.498229135614,8.51819193028669,66.4));
#97928=CARTESIAN_POINT('Ctrl Pts',(108.688075719542,8.08643077986812,66.8));
#97929=CARTESIAN_POINT('Ctrl Pts',(108.591215217539,8.30671708110066,66.594325014888));
#97930=CARTESIAN_POINT('Ctrl Pts',(108.498229135614,8.51819193028669,66.4));
#97931=CARTESIAN_POINT('',(108.184252771882,8.16622849545598,66.8));
#97932=CARTESIAN_POINT('Ctrl Pts',(108.498229135614,8.51819193028669,66.4));
#97933=CARTESIAN_POINT('Ctrl Pts',(108.344444794193,8.34580167649075,66.5943250148882));
#97934=CARTESIAN_POINT('Ctrl Pts',(108.184252771882,8.16622849545595,66.8));
#97935=CARTESIAN_POINT('',(107.153403786858,8.41371344057964,66.8));
#97936=CARTESIAN_POINT('Origin',(110.,18.,66.8));
#97937=CARTESIAN_POINT('',(107.033436854001,8.86985744356654,66.4));
#97938=CARTESIAN_POINT('Ctrl Pts',(107.153403786858,8.4137134405796,66.8));
#97939=CARTESIAN_POINT('Ctrl Pts',(107.092196168053,8.64643997271458,66.5943250148878));
#97940=CARTESIAN_POINT('Ctrl Pts',(107.033436854001,8.86985744356654,66.4));
#97941=CARTESIAN_POINT('',(106.668266848679,8.57134398716408,66.8));
#97942=CARTESIAN_POINT('Ctrl Pts',(107.033436854,8.86985744356654,66.4));
#97943=CARTESIAN_POINT('Ctrl Pts',(106.854578075882,8.72364677104165,66.5943250148884));
#97944=CARTESIAN_POINT('Ctrl Pts',(106.668266848679,8.57134398716406,66.8));
#97945=CARTESIAN_POINT('',(105.688824500252,8.97704229144512,66.8));
#97946=CARTESIAN_POINT('Origin',(110.,18.,66.8));
#97947=CARTESIAN_POINT('',(105.6416912025,9.44633736779169,66.4));
#97948=CARTESIAN_POINT('Ctrl Pts',(105.688824500252,8.97704229144508,66.8));
#97949=CARTESIAN_POINT('Ctrl Pts',(105.664776899358,9.21647855488566,66.5943250148881));
#97950=CARTESIAN_POINT('Ctrl Pts',(105.6416912025,9.44633736779169,66.4));
#97951=CARTESIAN_POINT('',(105.234319253049,9.20862428182348,66.8));
#97952=CARTESIAN_POINT('Ctrl Pts',(105.6416912025,9.44633736779169,66.4));
#97953=CARTESIAN_POINT('Ctrl Pts',(105.442162084401,9.32990646854146,66.5943250148875));
#97954=CARTESIAN_POINT('Ctrl Pts',(105.234319253049,9.20862428182346,66.8));
#97955=CARTESIAN_POINT('',(104.330400662421,9.76254630657499,66.8));
#97956=CARTESIAN_POINT('Origin',(110.,18.,66.8));
#97957=CARTESIAN_POINT('',(104.357261577992,10.2334368540005,66.4));
#97958=CARTESIAN_POINT('Ctrl Pts',(104.330400662421,9.76254630657495,66.8));
#97959=CARTESIAN_POINT('Ctrl Pts',(104.344105211182,10.0027965858725,66.5943250148878));
#97960=CARTESIAN_POINT('Ctrl Pts',(104.357261577992,10.2334368540005,66.4));
#97961=CARTESIAN_POINT('',(103.917718533797,10.0623774235676,66.8));
#97962=CARTESIAN_POINT('Ctrl Pts',(104.357261577992,10.2334368540005,66.4));
#97963=CARTESIAN_POINT('Ctrl Pts',(104.141975188998,10.1496526431757,66.5943250148879));
#97964=CARTESIAN_POINT('Ctrl Pts',(103.917718533797,10.0623774235676,66.8));
#97965=CARTESIAN_POINT('',(103.111581176602,10.7508837701784,66.8));
#97966=CARTESIAN_POINT('Origin',(110.,18.,66.8));
#97967=CARTESIAN_POINT('',(103.211774900609,11.2117749006092,66.4));
#97968=CARTESIAN_POINT('Ctrl Pts',(103.111581176602,10.7508837701784,66.8));
#97969=CARTESIAN_POINT('Ctrl Pts',(103.162700423544,10.9860323061103,66.5943250148885));
#97970=CARTESIAN_POINT('Ctrl Pts',(103.211774900609,11.2117749006092,66.4));
#97971=CARTESIAN_POINT('',(102.750883770178,11.1115811766025,66.8));
#97972=CARTESIAN_POINT('Ctrl Pts',(103.211774900609,11.2117749006092,66.4));
#97973=CARTESIAN_POINT('Ctrl Pts',(102.98603230611,11.1627004235442,66.5943250148886));
#97974=CARTESIAN_POINT('Ctrl Pts',(102.750883770178,11.1115811766025,66.8));
#97975=CARTESIAN_POINT('',(102.062377423568,11.9177185337975,66.8));
#97976=CARTESIAN_POINT('Origin',(110.,18.,66.8));
#97977=CARTESIAN_POINT('',(102.233436854001,12.3572615779923,66.4));
#97978=CARTESIAN_POINT('Ctrl Pts',(102.062377423568,11.9177185337975,66.8));
#97979=CARTESIAN_POINT('Ctrl Pts',(102.149652643177,12.1419751889998,66.5943250148859));
#97980=CARTESIAN_POINT('Ctrl Pts',(102.233436854001,12.3572615779923,66.4));
#97981=CARTESIAN_POINT('',(101.762546306575,12.3304006624208,66.8));
#97982=CARTESIAN_POINT('Ctrl Pts',(102.233436854001,12.3572615779923,66.4));
#97983=CARTESIAN_POINT('Ctrl Pts',(102.002796585872,12.3441052111816,66.594325014888));
#97984=CARTESIAN_POINT('Ctrl Pts',(101.762546306575,12.3304006624208,66.8));
#97985=CARTESIAN_POINT('',(101.208624281823,13.2343192530494,66.8));
#97986=CARTESIAN_POINT('Origin',(110.,18.,66.8));
#97987=CARTESIAN_POINT('',(101.446337367792,13.6416912025004,66.3999999999999));
#97988=CARTESIAN_POINT('Ctrl Pts',(101.208624281823,13.2343192530493,66.8));
#97989=CARTESIAN_POINT('Ctrl Pts',(101.329906468541,13.442162084401,66.5943250148876));
#97990=CARTESIAN_POINT('Ctrl Pts',(101.446337367792,13.6416912025004,66.3999999999999));
#97991=CARTESIAN_POINT('',(100.977042291445,13.6888245002517,66.8));
#97992=CARTESIAN_POINT('Ctrl Pts',(101.446337367792,13.6416912025004,66.3999999999999));
#97993=CARTESIAN_POINT('Ctrl Pts',(101.216478554886,13.6647768993583,66.5943250148876));
#97994=CARTESIAN_POINT('Ctrl Pts',(100.977042291445,13.6888245002517,66.8));
#97995=CARTESIAN_POINT('',(100.571343987164,14.6682668486788,66.8));
#97996=CARTESIAN_POINT('Origin',(110.,18.,66.8));
#97997=CARTESIAN_POINT('',(100.869857443567,15.0334368540005,66.4));
#97998=CARTESIAN_POINT('Ctrl Pts',(100.571343987164,14.6682668486787,66.8));
#97999=CARTESIAN_POINT('Ctrl Pts',(100.723646771041,14.8545780758816,66.5943250148891));
#98000=CARTESIAN_POINT('Ctrl Pts',(100.869857443567,15.0334368540005,66.4));
#98001=CARTESIAN_POINT('',(100.41371344058,15.1534037868576,66.8));
#98002=CARTESIAN_POINT('Ctrl Pts',(100.869857443567,15.0334368540005,66.4));
#98003=CARTESIAN_POINT('Ctrl Pts',(100.646439972716,15.092196168053,66.5943250148869));
#98004=CARTESIAN_POINT('Ctrl Pts',(100.41371344058,15.1534037868576,66.8));
#98005=CARTESIAN_POINT('',(100.166228495456,16.184252771882,66.8));
#98006=CARTESIAN_POINT('Origin',(110.,18.,66.8));
#98007=CARTESIAN_POINT('',(100.518191930287,16.4982291356138,66.4));
#98008=CARTESIAN_POINT('Ctrl Pts',(100.166228495456,16.184252771882,66.8));
#98009=CARTESIAN_POINT('Ctrl Pts',(100.345801676491,16.3444447941935,66.5943250148876));
#98010=CARTESIAN_POINT('Ctrl Pts',(100.518191930287,16.4982291356138,66.4));
#98011=CARTESIAN_POINT('',(100.086430779868,16.6880757195422,66.8));
#98012=CARTESIAN_POINT('Ctrl Pts',(100.518191930287,16.4982291356138,66.4));
#98013=CARTESIAN_POINT('Ctrl Pts',(100.306717081102,16.5912152175381,66.594325014887));
#98014=CARTESIAN_POINT('Ctrl Pts',(100.086430779868,16.6880757195423,66.8));
#98015=CARTESIAN_POINT('',(100.003253094606,17.7449484179612,66.8));
#98016=CARTESIAN_POINT('Origin',(110.,18.,66.8));
#98017=CARTESIAN_POINT('',(100.4,18.,66.4));
#98018=CARTESIAN_POINT('Ctrl Pts',(100.003253094606,17.7449484179611,66.8));
#98019=CARTESIAN_POINT('Ctrl Pts',(100.205674985111,17.8750767761431,66.5943250148885));
#98020=CARTESIAN_POINT('Ctrl Pts',(100.4,18.,66.4));
#98021=CARTESIAN_POINT('',(100.8,18.,66.));
#98022=CARTESIAN_POINT('',(100.4,18.,66.4));
#98023=CARTESIAN_POINT('Origin',(110.,18.,66.));
#98024=CARTESIAN_POINT('',(100.003253094606,18.2550515820388,66.8));
#98025=CARTESIAN_POINT('Ctrl Pts',(100.4,18.,66.4));
#98026=CARTESIAN_POINT('Ctrl Pts',(100.205674985111,18.1249232238571,66.5943250148889));
#98027=CARTESIAN_POINT('Ctrl Pts',(100.003253094606,18.2550515820389,66.8));
#98028=CARTESIAN_POINT('',(100.086430779868,19.3119242804578,66.8));
#98029=CARTESIAN_POINT('Origin',(110.,18.,66.8));
#98030=CARTESIAN_POINT('',(100.518191930287,19.5017708643862,66.4));
#98031=CARTESIAN_POINT('Ctrl Pts',(100.086430779868,19.3119242804577,66.8));
#98032=CARTESIAN_POINT('Ctrl Pts',(100.306717081101,19.4087847824617,66.5943250148874));
#98033=CARTESIAN_POINT('Ctrl Pts',(100.518191930287,19.5017708643862,66.4));
#98034=CARTESIAN_POINT('',(100.166228495456,19.815747228118,66.8));
#98035=CARTESIAN_POINT('Ctrl Pts',(100.518191930287,19.5017708643862,66.4));
#98036=CARTESIAN_POINT('Ctrl Pts',(100.345801676492,19.6555552058062,66.5943250148871));
#98037=CARTESIAN_POINT('Ctrl Pts',(100.166228495456,19.815747228118,66.8));
#98038=CARTESIAN_POINT('',(100.41371344058,20.8465962131424,66.8));
#98039=CARTESIAN_POINT('Origin',(110.,18.,66.8));
#98040=CARTESIAN_POINT('',(100.869857443567,20.9665631459995,66.4));
#98041=CARTESIAN_POINT('Ctrl Pts',(100.41371344058,20.8465962131424,66.8));
#98042=CARTESIAN_POINT('Ctrl Pts',(100.646439972714,20.9078038319467,66.5943250148879));
#98043=CARTESIAN_POINT('Ctrl Pts',(100.869857443567,20.9665631459995,66.4));
#98044=CARTESIAN_POINT('',(100.571343987164,21.3317331513213,66.8));
#98045=CARTESIAN_POINT('Ctrl Pts',(100.869857443567,20.9665631459995,66.4));
#98046=CARTESIAN_POINT('Ctrl Pts',(100.723646771042,21.1454219241175,66.594325014888));
#98047=CARTESIAN_POINT('Ctrl Pts',(100.571343987164,21.3317331513213,66.8));
#98048=CARTESIAN_POINT('',(100.977042291445,22.3111754997483,66.8));
#98049=CARTESIAN_POINT('Origin',(110.,18.,66.8));
#98050=CARTESIAN_POINT('',(101.446337367792,22.3583087974996,66.3999999999999));
#98051=CARTESIAN_POINT('Ctrl Pts',(100.977042291445,22.3111754997483,66.8));
#98052=CARTESIAN_POINT('Ctrl Pts',(101.216478554886,22.3352231006417,66.5943250148875));
#98053=CARTESIAN_POINT('Ctrl Pts',(101.446337367792,22.3583087974996,66.3999999999999));
#98054=CARTESIAN_POINT('',(101.208624281823,22.7656807469507,66.8));
#98055=CARTESIAN_POINT('Ctrl Pts',(101.446337367792,22.3583087974996,66.3999999999999));
#98056=CARTESIAN_POINT('Ctrl Pts',(101.329906468541,22.5578379155989,66.5943250148875));
#98057=CARTESIAN_POINT('Ctrl Pts',(101.208624281823,22.7656807469507,66.8));
#98058=CARTESIAN_POINT('',(101.762546306575,23.6695993375792,66.8));
#98059=CARTESIAN_POINT('Origin',(110.,18.,66.8));
#98060=CARTESIAN_POINT('',(102.233436854001,23.6427384220077,66.4));
#98061=CARTESIAN_POINT('Ctrl Pts',(101.762546306575,23.6695993375792,66.8));
#98062=CARTESIAN_POINT('Ctrl Pts',(102.002796585873,23.6558947888183,66.5943250148876));
#98063=CARTESIAN_POINT('Ctrl Pts',(102.233436854001,23.6427384220077,66.4));
#98064=CARTESIAN_POINT('',(102.062377423568,24.0822814662025,66.8));
#98065=CARTESIAN_POINT('Ctrl Pts',(102.233436854001,23.6427384220077,66.4));
#98066=CARTESIAN_POINT('Ctrl Pts',(102.149652643175,23.858024811003,66.5943250148884));
#98067=CARTESIAN_POINT('Ctrl Pts',(102.062377423568,24.0822814662026,66.8));
#98068=CARTESIAN_POINT('',(102.750883770178,24.8884188233975,66.8));
#98069=CARTESIAN_POINT('Origin',(110.,18.,66.8));
#98070=CARTESIAN_POINT('',(103.211774900609,24.7882250993908,66.4));
#98071=CARTESIAN_POINT('Ctrl Pts',(102.750883770178,24.8884188233975,66.8));
#98072=CARTESIAN_POINT('Ctrl Pts',(102.986032306111,24.8372995764558,66.5943250148883));
#98073=CARTESIAN_POINT('Ctrl Pts',(103.211774900609,24.7882250993908,66.4));
#98074=CARTESIAN_POINT('',(103.111581176602,25.2491162298216,66.8));
#98075=CARTESIAN_POINT('Ctrl Pts',(103.211774900609,24.7882250993908,66.4));
#98076=CARTESIAN_POINT('Ctrl Pts',(103.162700423544,25.0139676938896,66.5943250148885));
#98077=CARTESIAN_POINT('Ctrl Pts',(103.111581176602,25.2491162298216,66.8));
#98078=CARTESIAN_POINT('',(103.917718533797,25.9376225764324,66.8));
#98079=CARTESIAN_POINT('Origin',(110.,18.,66.8));
#98080=CARTESIAN_POINT('',(104.357261577992,25.7665631459995,66.4));
#98081=CARTESIAN_POINT('Ctrl Pts',(103.917718533797,25.9376225764324,66.8));
#98082=CARTESIAN_POINT('Ctrl Pts',(104.141975188999,25.8503473568237,66.5943250148866));
#98083=CARTESIAN_POINT('Ctrl Pts',(104.357261577992,25.7665631459995,66.4));
#98084=CARTESIAN_POINT('',(104.330400662421,26.237453693425,66.8));
#98085=CARTESIAN_POINT('Ctrl Pts',(104.357261577992,25.7665631459995,66.4));
#98086=CARTESIAN_POINT('Ctrl Pts',(104.344105211182,25.9972034141269,66.5943250148872));
#98087=CARTESIAN_POINT('Ctrl Pts',(104.330400662421,26.237453693425,66.8));
#98088=CARTESIAN_POINT('',(105.234319253049,26.7913757181765,66.8));
#98089=CARTESIAN_POINT('Origin',(110.,18.,66.8));
#98090=CARTESIAN_POINT('',(105.6416912025,26.5536626322083,66.4));
#98091=CARTESIAN_POINT('Ctrl Pts',(105.234319253049,26.7913757181765,66.8));
#98092=CARTESIAN_POINT('Ctrl Pts',(105.4421620844,26.670093531459,66.5943250148883));
#98093=CARTESIAN_POINT('Ctrl Pts',(105.6416912025,26.5536626322083,66.3999999999999));
#98094=CARTESIAN_POINT('',(105.688824500252,27.0229577085549,66.8));
#98095=CARTESIAN_POINT('Ctrl Pts',(105.6416912025,26.5536626322083,66.4));
#98096=CARTESIAN_POINT('Ctrl Pts',(105.664776899358,26.7835214451143,66.594325014888));
#98097=CARTESIAN_POINT('Ctrl Pts',(105.688824500252,27.0229577085549,66.8));
#98098=CARTESIAN_POINT('',(106.668266848679,27.4286560128359,66.8));
#98099=CARTESIAN_POINT('Origin',(110.,18.,66.8));
#98100=CARTESIAN_POINT('',(107.033436854,27.1301425564335,66.4));
#98101=CARTESIAN_POINT('Ctrl Pts',(106.668266848679,27.4286560128359,66.8));
#98102=CARTESIAN_POINT('Ctrl Pts',(106.854578075883,27.2763532289579,66.5943250148878));
#98103=CARTESIAN_POINT('Ctrl Pts',(107.033436854,27.1301425564335,66.4));
#98104=CARTESIAN_POINT('',(107.153403786858,27.5862865594204,66.8));
#98105=CARTESIAN_POINT('Ctrl Pts',(107.033436854,27.1301425564335,66.4));
#98106=CARTESIAN_POINT('Ctrl Pts',(107.092196168053,27.3535600272857,66.594325014888));
#98107=CARTESIAN_POINT('Ctrl Pts',(107.153403786858,27.5862865594204,66.8));
#98108=CARTESIAN_POINT('',(108.184252771882,27.833771504544,66.8));
#98109=CARTESIAN_POINT('Origin',(110.,18.,66.8));
#98110=CARTESIAN_POINT('',(108.498229135614,27.4818080697133,66.4));
#98111=CARTESIAN_POINT('Ctrl Pts',(108.184252771882,27.833771504544,66.8));
#98112=CARTESIAN_POINT('Ctrl Pts',(108.344444794194,27.6541983235085,66.5943250148873));
#98113=CARTESIAN_POINT('Ctrl Pts',(108.498229135614,27.4818080697133,66.4));
#98114=CARTESIAN_POINT('',(108.688075719542,27.9135692201318,66.8));
#98115=CARTESIAN_POINT('Ctrl Pts',(108.498229135614,27.4818080697133,66.4));
#98116=CARTESIAN_POINT('Ctrl Pts',(108.591215217538,27.6932829188985,66.5943250148872));
#98117=CARTESIAN_POINT('Ctrl Pts',(108.688075719542,27.9135692201319,66.8));
#98118=CARTESIAN_POINT('',(109.744948417961,27.9967469053937,66.8));
#98119=CARTESIAN_POINT('Origin',(110.,18.,66.8));
#98120=CARTESIAN_POINT('',(110.,27.6,66.4));
#98121=CARTESIAN_POINT('Ctrl Pts',(109.744948417961,27.9967469053938,66.8));
#98122=CARTESIAN_POINT('Ctrl Pts',(109.875076776144,27.794325014887,66.594325014887));
#98123=CARTESIAN_POINT('Ctrl Pts',(110.,27.6,66.4));
#98124=CARTESIAN_POINT('',(110.255051582039,27.9967469053937,66.8));
#98125=CARTESIAN_POINT('Ctrl Pts',(110.,27.6,66.4));
#98126=CARTESIAN_POINT('Ctrl Pts',(110.124923223856,27.7943250148865,66.5943250148864));
#98127=CARTESIAN_POINT('Ctrl Pts',(110.255051582039,27.9967469053937,66.8));
#98128=CARTESIAN_POINT('',(111.311924280458,27.9135692201318,66.8));
#98129=CARTESIAN_POINT('Origin',(110.,18.,66.8));
#98130=CARTESIAN_POINT('',(111.501770864386,27.4818080697133,66.4));
#98131=CARTESIAN_POINT('Ctrl Pts',(111.311924280458,27.9135692201318,66.8));
#98132=CARTESIAN_POINT('Ctrl Pts',(111.408784782462,27.693282918898,66.5943250148868));
#98133=CARTESIAN_POINT('Ctrl Pts',(111.501770864386,27.4818080697133,66.4));
#98134=CARTESIAN_POINT('',(111.815747228118,27.833771504544,66.8));
#98135=CARTESIAN_POINT('Ctrl Pts',(111.501770864386,27.4818080697133,66.4));
#98136=CARTESIAN_POINT('Ctrl Pts',(111.655555205806,27.6541983235077,66.5943250148865));
#98137=CARTESIAN_POINT('Ctrl Pts',(111.815747228118,27.833771504544,66.8));
#98138=CARTESIAN_POINT('',(112.846596213142,27.5862865594204,66.8));
#98139=CARTESIAN_POINT('Origin',(110.,18.,66.8));
#98140=CARTESIAN_POINT('',(112.966563146,27.1301425564335,66.4));
#98141=CARTESIAN_POINT('Ctrl Pts',(112.846596213142,27.5862865594204,66.8));
#98142=CARTESIAN_POINT('Ctrl Pts',(112.907803831947,27.3535600272835,66.5943250148861));
#98143=CARTESIAN_POINT('Ctrl Pts',(112.966563146,27.1301425564335,66.4));
#98144=CARTESIAN_POINT('',(113.331733151321,27.4286560128359,66.8));
#98145=CARTESIAN_POINT('Ctrl Pts',(112.966563146,27.1301425564335,66.4));
#98146=CARTESIAN_POINT('Ctrl Pts',(113.145421924116,27.2763532289572,66.5943250148869));
#98147=CARTESIAN_POINT('Ctrl Pts',(113.331733151321,27.4286560128359,66.8));
#98148=CARTESIAN_POINT('',(114.311175499748,27.0229577085549,66.8));
#98149=CARTESIAN_POINT('Origin',(110.,18.,66.8));
#98150=CARTESIAN_POINT('',(114.3583087975,26.5536626322083,66.4));
#98151=CARTESIAN_POINT('Ctrl Pts',(114.311175499748,27.0229577085549,66.8));
#98152=CARTESIAN_POINT('Ctrl Pts',(114.335223100642,26.7835214451131,66.594325014887));
#98153=CARTESIAN_POINT('Ctrl Pts',(114.3583087975,26.5536626322083,66.4));
#98154=CARTESIAN_POINT('',(114.765680746951,26.7913757181765,66.8));
#98155=CARTESIAN_POINT('Ctrl Pts',(114.3583087975,26.5536626322083,66.4));
#98156=CARTESIAN_POINT('Ctrl Pts',(114.557837915598,26.6700935314582,66.594325014887));
#98157=CARTESIAN_POINT('Ctrl Pts',(114.765680746951,26.7913757181765,66.8));
#98158=CARTESIAN_POINT('',(115.669599337579,26.237453693425,66.8));
#98159=CARTESIAN_POINT('Origin',(110.,18.,66.8));
#98160=CARTESIAN_POINT('',(115.642738422008,25.7665631459995,66.4));
#98161=CARTESIAN_POINT('Ctrl Pts',(115.669599337579,26.237453693425,66.8));
#98162=CARTESIAN_POINT('Ctrl Pts',(115.655894788818,25.9972034141256,66.5943250148862));
#98163=CARTESIAN_POINT('Ctrl Pts',(115.642738422008,25.7665631459995,66.4));
#98164=CARTESIAN_POINT('',(116.082281466203,25.9376225764324,66.8));
#98165=CARTESIAN_POINT('Ctrl Pts',(115.642738422008,25.7665631459995,66.4));
#98166=CARTESIAN_POINT('Ctrl Pts',(115.858024811,25.8503473568235,66.5943250148862));
#98167=CARTESIAN_POINT('Ctrl Pts',(116.082281466202,25.9376225764324,66.8));
#98168=CARTESIAN_POINT('',(116.888418823398,25.2491162298216,66.8));
#98169=CARTESIAN_POINT('Origin',(110.,18.,66.8));
#98170=CARTESIAN_POINT('',(116.788225099391,24.7882250993908,66.4));
#98171=CARTESIAN_POINT('Ctrl Pts',(116.888418823398,25.2491162298216,66.8));
#98172=CARTESIAN_POINT('Ctrl Pts',(116.837299576455,25.0139676938873,66.5943250148865));
#98173=CARTESIAN_POINT('Ctrl Pts',(116.788225099391,24.7882250993908,66.4));
#98174=CARTESIAN_POINT('',(117.249116229822,24.8884188233975,66.8));
#98175=CARTESIAN_POINT('Ctrl Pts',(116.788225099391,24.7882250993908,66.4));
#98176=CARTESIAN_POINT('Ctrl Pts',(117.013967693887,24.8372995764551,66.5943250148859));
#98177=CARTESIAN_POINT('Ctrl Pts',(117.249116229822,24.8884188233975,66.8));
#98178=CARTESIAN_POINT('',(117.937622576432,24.0822814662025,66.8));
#98179=CARTESIAN_POINT('Origin',(110.,18.,66.8));
#98180=CARTESIAN_POINT('',(117.766563145999,23.6427384220077,66.4));
#98181=CARTESIAN_POINT('Ctrl Pts',(117.937622576432,24.0822814662025,66.8));
#98182=CARTESIAN_POINT('Ctrl Pts',(117.850347356824,23.8580248110013,66.5943250148869));
#98183=CARTESIAN_POINT('Ctrl Pts',(117.766563146,23.6427384220077,66.4));
#98184=CARTESIAN_POINT('',(118.237453693425,23.6695993375792,66.8));
#98185=CARTESIAN_POINT('Ctrl Pts',(117.766563145999,23.6427384220077,66.4));
#98186=CARTESIAN_POINT('Ctrl Pts',(117.997203414128,23.6558947888183,66.5943250148878));
#98187=CARTESIAN_POINT('Ctrl Pts',(118.237453693425,23.6695993375792,66.8));
#98188=CARTESIAN_POINT('',(118.791375718177,22.7656807469507,66.8));
#98189=CARTESIAN_POINT('Origin',(110.,18.,66.8));
#98190=CARTESIAN_POINT('',(118.553662632208,22.3583087974996,66.4));
#98191=CARTESIAN_POINT('Ctrl Pts',(118.791375718177,22.7656807469507,66.8));
#98192=CARTESIAN_POINT('Ctrl Pts',(118.670093531458,22.5578379155986,66.5943250148872));
#98193=CARTESIAN_POINT('Ctrl Pts',(118.553662632208,22.3583087974996,66.4));
#98194=CARTESIAN_POINT('',(119.022957708555,22.3111754997483,66.8));
#98195=CARTESIAN_POINT('Ctrl Pts',(118.553662632208,22.3583087974996,66.4));
#98196=CARTESIAN_POINT('Ctrl Pts',(118.783521445112,22.3352231006419,66.5943250148863));
#98197=CARTESIAN_POINT('Ctrl Pts',(119.022957708555,22.3111754997483,66.8));
#98198=CARTESIAN_POINT('',(119.428656012836,21.3317331513213,66.8));
#98199=CARTESIAN_POINT('Origin',(110.,18.,66.8));
#98200=CARTESIAN_POINT('',(119.130142556433,20.9665631459995,66.4));
#98201=CARTESIAN_POINT('Ctrl Pts',(119.428656012836,21.3317331513213,66.8));
#98202=CARTESIAN_POINT('Ctrl Pts',(119.276353228957,21.145421924116,66.5943250148865));
#98203=CARTESIAN_POINT('Ctrl Pts',(119.130142556433,20.9665631459995,66.4));
#98204=CARTESIAN_POINT('',(119.58628655942,20.8465962131424,66.8));
#98205=CARTESIAN_POINT('Ctrl Pts',(119.130142556433,20.9665631459995,66.4));
#98206=CARTESIAN_POINT('Ctrl Pts',(119.353560027284,20.9078038319471,66.5943250148866));
#98207=CARTESIAN_POINT('Ctrl Pts',(119.58628655942,20.8465962131424,66.8));
#98208=CARTESIAN_POINT('',(119.833771504544,19.815747228118,66.8));
#98209=CARTESIAN_POINT('Origin',(110.,18.,66.8));
#98210=CARTESIAN_POINT('',(119.481808069713,19.5017708643862,66.4));
#98211=CARTESIAN_POINT('Ctrl Pts',(119.833771504544,19.815747228118,66.8));
#98212=CARTESIAN_POINT('Ctrl Pts',(119.654198323508,19.6555552058055,66.5943250148863));
#98213=CARTESIAN_POINT('Ctrl Pts',(119.481808069713,19.5017708643862,66.4));
#98214=CARTESIAN_POINT('',(119.913569220132,19.3119242804578,66.8));
#98215=CARTESIAN_POINT('Ctrl Pts',(119.481808069713,19.5017708643862,66.4));
#98216=CARTESIAN_POINT('Ctrl Pts',(119.693282918898,19.4087847824621,66.5943250148865));
#98217=CARTESIAN_POINT('Ctrl Pts',(119.913569220132,19.3119242804577,66.8));
#98218=CARTESIAN_POINT('',(119.996746905394,18.2550515820388,66.8));
#98219=CARTESIAN_POINT('Origin',(110.,18.,66.8));
#98220=CARTESIAN_POINT('',(119.6,18.,66.4));
#98221=CARTESIAN_POINT('Ctrl Pts',(119.996746905394,18.2550515820388,66.8));
#98222=CARTESIAN_POINT('Ctrl Pts',(119.794325014887,18.1249232238558,66.5943250148867));
#98223=CARTESIAN_POINT('Ctrl Pts',(119.6,18.,66.4));
#98224=CARTESIAN_POINT('',(119.996746905394,17.7449484179612,66.8));
#98225=CARTESIAN_POINT('Ctrl Pts',(119.6,18.,66.4));
#98226=CARTESIAN_POINT('Ctrl Pts',(119.794325014887,17.8750767761443,66.5943250148866));
#98227=CARTESIAN_POINT('Ctrl Pts',(119.996746905394,17.7449484179612,66.8));
#98228=CARTESIAN_POINT('Origin',(110.,18.,66.8));
#98229=CARTESIAN_POINT('Origin',(110.,18.,73.5));
#98230=CARTESIAN_POINT('',(119.58628655942,15.1534037868576,80.2));
#98231=CARTESIAN_POINT('Origin',(110.,18.,80.2));
#98232=CARTESIAN_POINT('',(119.58628655942,15.1534037868576,73.5));
#98233=CARTESIAN_POINT('Origin',(110.,18.,73.5));
#98234=CARTESIAN_POINT('',(119.996746905394,17.7449484179612,80.2));
#98235=CARTESIAN_POINT('',(119.996746905394,17.7449484179612,73.5));
#98236=CARTESIAN_POINT('Origin',(110.,18.,80.2));
#98237=CARTESIAN_POINT('Origin',(119.656824470371,14.3891495256052,81.));
#98238=CARTESIAN_POINT('',(119.130142556433,15.0334368540005,80.6));
#98239=CARTESIAN_POINT('',(119.130142556433,15.0334368540005,81.));
#98240=CARTESIAN_POINT('',(119.428656012836,14.6682668486787,80.2));
#98241=CARTESIAN_POINT('Ctrl Pts',(119.428656012836,14.6682668486787,80.2));
#98242=CARTESIAN_POINT('Ctrl Pts',(119.276353228957,14.8545780758837,80.4056749851132));
#98243=CARTESIAN_POINT('Ctrl Pts',(119.130142556433,15.0334368540005,80.6));
#98244=CARTESIAN_POINT('',(119.428656012836,14.6682668486787,73.5));
#98245=CARTESIAN_POINT('Origin',(119.130142556433,15.0334368540005,81.));
#98246=CARTESIAN_POINT('Ctrl Pts',(119.130142556433,15.0334368540005,80.6));
#98247=CARTESIAN_POINT('Ctrl Pts',(119.353560027284,15.092196168053,80.4056749851132));
#98248=CARTESIAN_POINT('Ctrl Pts',(119.58628655942,15.1534037868576,80.2));
#98249=CARTESIAN_POINT('Origin',(110.,18.,73.5));
#98250=CARTESIAN_POINT('',(119.022957708555,13.6888245002517,80.2));
#98251=CARTESIAN_POINT('Origin',(110.,18.,80.2));
#98252=CARTESIAN_POINT('',(119.022957708555,13.6888245002517,73.5));
#98253=CARTESIAN_POINT('Origin',(110.,18.,80.6));
#98254=CARTESIAN_POINT('',(100.8,18.,81.));
#98255=CARTESIAN_POINT('Origin',(110.,18.,81.));
#98256=CARTESIAN_POINT('',(100.4,18.,80.6));
#98257=CARTESIAN_POINT('',(100.4,18.,80.6));
#98258=CARTESIAN_POINT('',(100.003253094606,17.7449484179612,80.2));
#98259=CARTESIAN_POINT('Ctrl Pts',(100.4,18.,80.6));
#98260=CARTESIAN_POINT('Ctrl Pts',(100.205674985113,17.8750767761442,80.4056749851132));
#98261=CARTESIAN_POINT('Ctrl Pts',(100.003253094606,17.7449484179612,80.2));
#98262=CARTESIAN_POINT('',(100.086430779868,16.6880757195422,80.2));
#98263=CARTESIAN_POINT('Origin',(110.,18.,80.2));
#98264=CARTESIAN_POINT('',(100.518191930287,16.4982291356138,80.6));
#98265=CARTESIAN_POINT('Ctrl Pts',(100.086430779868,16.6880757195422,80.2));
#98266=CARTESIAN_POINT('Ctrl Pts',(100.306717081103,16.5912152175373,80.4056749851144));
#98267=CARTESIAN_POINT('Ctrl Pts',(100.518191930287,16.4982291356138,80.6));
#98268=CARTESIAN_POINT('',(100.166228495456,16.184252771882,80.2));
#98269=CARTESIAN_POINT('Ctrl Pts',(100.518191930287,16.4982291356138,80.6));
#98270=CARTESIAN_POINT('Ctrl Pts',(100.345801676493,16.3444447941946,80.4056749851138));
#98271=CARTESIAN_POINT('Ctrl Pts',(100.166228495456,16.184252771882,80.2));
#98272=CARTESIAN_POINT('',(100.41371344058,15.1534037868576,80.2));
#98273=CARTESIAN_POINT('Origin',(110.,18.,80.2));
#98274=CARTESIAN_POINT('',(100.869857443567,15.0334368540005,80.6));
#98275=CARTESIAN_POINT('Ctrl Pts',(100.41371344058,15.1534037868576,80.2));
#98276=CARTESIAN_POINT('Ctrl Pts',(100.646439972715,15.0921961680531,80.4056749851129));
#98277=CARTESIAN_POINT('Ctrl Pts',(100.869857443567,15.0334368540005,80.6));
#98278=CARTESIAN_POINT('',(100.571343987164,14.6682668486788,80.2));
#98279=CARTESIAN_POINT('Ctrl Pts',(100.869857443567,15.0334368540005,80.6));
#98280=CARTESIAN_POINT('Ctrl Pts',(100.723646771043,14.854578075884,80.4056749851136));
#98281=CARTESIAN_POINT('Ctrl Pts',(100.571343987164,14.6682668486787,80.2));
#98282=CARTESIAN_POINT('',(100.977042291445,13.6888245002517,80.2));
#98283=CARTESIAN_POINT('Origin',(110.,18.,80.2));
#98284=CARTESIAN_POINT('',(101.446337367792,13.6416912025004,80.6));
#98285=CARTESIAN_POINT('Ctrl Pts',(100.977042291445,13.6888245002517,80.2));
#98286=CARTESIAN_POINT('Ctrl Pts',(101.216478554888,13.6647768993581,80.405674985114));
#98287=CARTESIAN_POINT('Ctrl Pts',(101.446337367792,13.6416912025004,80.6));
#98288=CARTESIAN_POINT('',(101.208624281823,13.2343192530494,80.2));
#98289=CARTESIAN_POINT('Ctrl Pts',(101.446337367792,13.6416912025004,80.6));
#98290=CARTESIAN_POINT('Ctrl Pts',(101.329906468542,13.4421620844021,80.4056749851134));
#98291=CARTESIAN_POINT('Ctrl Pts',(101.208624281823,13.2343192530494,80.2));
#98292=CARTESIAN_POINT('',(101.762546306575,12.3304006624208,80.2));
#98293=CARTESIAN_POINT('Origin',(110.,18.,80.2));
#98294=CARTESIAN_POINT('',(102.233436854001,12.3572615779923,80.6));
#98295=CARTESIAN_POINT('Ctrl Pts',(101.762546306575,12.3304006624208,80.2));
#98296=CARTESIAN_POINT('Ctrl Pts',(102.002796585874,12.3441052111818,80.4056749851137));
#98297=CARTESIAN_POINT('Ctrl Pts',(102.233436854001,12.3572615779923,80.6));
#98298=CARTESIAN_POINT('',(102.062377423568,11.9177185337975,80.2));
#98299=CARTESIAN_POINT('Ctrl Pts',(102.233436854001,12.3572615779923,80.6));
#98300=CARTESIAN_POINT('Ctrl Pts',(102.149652643177,12.1419751889997,80.405674985114));
#98301=CARTESIAN_POINT('Ctrl Pts',(102.062377423568,11.9177185337975,80.2));
#98302=CARTESIAN_POINT('',(102.750883770178,11.1115811766025,80.2));
#98303=CARTESIAN_POINT('Origin',(110.,18.,80.2));
#98304=CARTESIAN_POINT('',(103.211774900609,11.2117749006092,80.6));
#98305=CARTESIAN_POINT('Ctrl Pts',(102.750883770178,11.1115811766025,80.2));
#98306=CARTESIAN_POINT('Ctrl Pts',(102.986032306113,11.1627004235447,80.4056749851135));
#98307=CARTESIAN_POINT('Ctrl Pts',(103.211774900609,11.2117749006092,80.6));
#98308=CARTESIAN_POINT('',(103.111581176602,10.7508837701784,80.2));
#98309=CARTESIAN_POINT('Ctrl Pts',(103.211774900609,11.2117749006092,80.6));
#98310=CARTESIAN_POINT('Ctrl Pts',(103.162700423545,10.9860323061126,80.4056749851134));
#98311=CARTESIAN_POINT('Ctrl Pts',(103.111581176602,10.7508837701784,80.2));
#98312=CARTESIAN_POINT('',(103.917718533797,10.0623774235676,80.2));
#98313=CARTESIAN_POINT('Origin',(110.,18.,80.2));
#98314=CARTESIAN_POINT('',(104.357261577992,10.2334368540005,80.6));
#98315=CARTESIAN_POINT('Ctrl Pts',(103.917718533797,10.0623774235676,80.2));
#98316=CARTESIAN_POINT('Ctrl Pts',(104.141975188999,10.1496526431763,80.4056749851136));
#98317=CARTESIAN_POINT('Ctrl Pts',(104.357261577992,10.2334368540005,80.6));
#98318=CARTESIAN_POINT('',(104.330400662421,9.76254630657499,80.2));
#98319=CARTESIAN_POINT('Ctrl Pts',(104.357261577992,10.2334368540005,80.6));
#98320=CARTESIAN_POINT('Ctrl Pts',(104.344105211182,10.0027965858746,80.4056749851139));
#98321=CARTESIAN_POINT('Ctrl Pts',(104.330400662421,9.76254630657499,80.2));
#98322=CARTESIAN_POINT('',(105.234319253049,9.20862428182348,80.2));
#98323=CARTESIAN_POINT('Origin',(110.,18.,80.2));
#98324=CARTESIAN_POINT('',(105.6416912025,9.44633736779169,80.6));
#98325=CARTESIAN_POINT('Ctrl Pts',(105.234319253049,9.20862428182348,80.2));
#98326=CARTESIAN_POINT('Ctrl Pts',(105.442162084402,9.32990646854195,80.4056749851133));
#98327=CARTESIAN_POINT('Ctrl Pts',(105.6416912025,9.44633736779169,80.6));
#98328=CARTESIAN_POINT('',(105.688824500252,8.97704229144512,80.2));
#98329=CARTESIAN_POINT('Ctrl Pts',(105.6416912025,9.44633736779169,80.6));
#98330=CARTESIAN_POINT('Ctrl Pts',(105.664776899358,9.21647855488777,80.4056749851137));
#98331=CARTESIAN_POINT('Ctrl Pts',(105.688824500252,8.97704229144512,80.2));
#98332=CARTESIAN_POINT('',(106.668266848679,8.57134398716408,80.2));
#98333=CARTESIAN_POINT('Origin',(110.,18.,80.2));
#98334=CARTESIAN_POINT('',(107.033436854001,8.86985744356654,80.6));
#98335=CARTESIAN_POINT('Ctrl Pts',(106.668266848679,8.57134398716408,80.2));
#98336=CARTESIAN_POINT('Ctrl Pts',(106.854578075884,8.72364677104273,80.4056749851131));
#98337=CARTESIAN_POINT('Ctrl Pts',(107.033436854001,8.86985744356654,80.6));
#98338=CARTESIAN_POINT('',(107.153403786858,8.41371344057964,80.2));
#98339=CARTESIAN_POINT('Ctrl Pts',(107.033436854001,8.86985744356654,80.6));
#98340=CARTESIAN_POINT('Ctrl Pts',(107.092196168053,8.64643997271655,80.4056749851139));
#98341=CARTESIAN_POINT('Ctrl Pts',(107.153403786858,8.41371344057964,80.2));
#98342=CARTESIAN_POINT('',(108.184252771882,8.16622849545598,80.2));
#98343=CARTESIAN_POINT('Origin',(110.,18.,80.2));
#98344=CARTESIAN_POINT('',(108.498229135614,8.51819193028669,80.6));
#98345=CARTESIAN_POINT('Ctrl Pts',(108.184252771882,8.16622849545598,80.2));
#98346=CARTESIAN_POINT('Ctrl Pts',(108.344444794194,8.34580167649242,80.4056749851137));
#98347=CARTESIAN_POINT('Ctrl Pts',(108.498229135614,8.51819193028669,80.6));
#98348=CARTESIAN_POINT('',(108.688075719542,8.08643077986816,80.2));
#98349=CARTESIAN_POINT('Ctrl Pts',(108.498229135614,8.51819193028669,80.6));
#98350=CARTESIAN_POINT('Ctrl Pts',(108.591215217538,8.30671708110244,80.4056749851136));
#98351=CARTESIAN_POINT('Ctrl Pts',(108.688075719542,8.08643077986816,80.2));
#98352=CARTESIAN_POINT('',(109.744948417961,8.00325309460625,80.2));
#98353=CARTESIAN_POINT('Origin',(110.,18.,80.2));
#98354=CARTESIAN_POINT('',(110.,8.40000000000002,80.6));
#98355=CARTESIAN_POINT('Ctrl Pts',(109.744948417961,8.00325309460625,80.2));
#98356=CARTESIAN_POINT('Ctrl Pts',(109.875076776144,8.20567498511359,80.4056749851136));
#98357=CARTESIAN_POINT('Ctrl Pts',(110.,8.40000000000002,80.6));
#98358=CARTESIAN_POINT('',(110.255051582039,8.00325309460625,80.2));
#98359=CARTESIAN_POINT('Ctrl Pts',(110.,8.40000000000002,80.6));
#98360=CARTESIAN_POINT('Ctrl Pts',(110.124923223856,8.20567498511304,80.405674985113));
#98361=CARTESIAN_POINT('Ctrl Pts',(110.255051582039,8.00325309460625,80.2));
#98362=CARTESIAN_POINT('',(111.311924280458,8.08643077986816,80.2));
#98363=CARTESIAN_POINT('Origin',(110.,18.,80.2));
#98364=CARTESIAN_POINT('',(111.501770864386,8.51819193028669,80.6));
#98365=CARTESIAN_POINT('Ctrl Pts',(111.311924280458,8.08643077986816,80.2));
#98366=CARTESIAN_POINT('Ctrl Pts',(111.408784782462,8.30671708110237,80.4056749851135));
#98367=CARTESIAN_POINT('Ctrl Pts',(111.501770864386,8.51819193028669,80.6));
#98368=CARTESIAN_POINT('',(111.815747228118,8.16622849545598,80.2));
#98369=CARTESIAN_POINT('Ctrl Pts',(111.501770864386,8.51819193028669,80.6));
#98370=CARTESIAN_POINT('Ctrl Pts',(111.655555205805,8.34580167649278,80.4056749851141));
#98371=CARTESIAN_POINT('Ctrl Pts',(111.815747228118,8.16622849545598,80.2));
#98372=CARTESIAN_POINT('',(112.846596213142,8.41371344057965,80.2));
#98373=CARTESIAN_POINT('Origin',(110.,18.,80.2));
#98374=CARTESIAN_POINT('',(112.966563146,8.86985744356654,80.6));
#98375=CARTESIAN_POINT('Ctrl Pts',(112.846596213142,8.41371344057965,80.2));
#98376=CARTESIAN_POINT('Ctrl Pts',(112.907803831947,8.64643997271638,80.4056749851138));
#98377=CARTESIAN_POINT('Ctrl Pts',(112.966563146,8.86985744356654,80.6));
#98378=CARTESIAN_POINT('',(113.331733151321,8.57134398716408,80.2));
#98379=CARTESIAN_POINT('Ctrl Pts',(112.966563146,8.86985744356654,80.6));
#98380=CARTESIAN_POINT('Ctrl Pts',(113.145421924116,8.72364677104327,80.4056749851138));
#98381=CARTESIAN_POINT('Ctrl Pts',(113.331733151321,8.57134398716408,80.2));
#98382=CARTESIAN_POINT('',(114.311175499748,8.97704229144512,80.2));
#98383=CARTESIAN_POINT('Origin',(110.,18.,80.2));
#98384=CARTESIAN_POINT('',(114.3583087975,9.44633736779169,80.6));
#98385=CARTESIAN_POINT('Ctrl Pts',(114.311175499748,8.97704229144512,80.2));
#98386=CARTESIAN_POINT('Ctrl Pts',(114.335223100642,9.21647855488781,80.4056749851138));
#98387=CARTESIAN_POINT('Ctrl Pts',(114.3583087975,9.44633736779169,80.6));
#98388=CARTESIAN_POINT('',(114.765680746951,9.20862428182348,80.2));
#98389=CARTESIAN_POINT('Ctrl Pts',(114.3583087975,9.44633736779169,80.6));
#98390=CARTESIAN_POINT('Ctrl Pts',(114.557837915597,9.32990646854248,80.4056749851141));
#98391=CARTESIAN_POINT('Ctrl Pts',(114.765680746951,9.20862428182348,80.2));
#98392=CARTESIAN_POINT('',(115.669599337579,9.762546306575,80.2));
#98393=CARTESIAN_POINT('Origin',(110.,18.,80.2));
#98394=CARTESIAN_POINT('',(115.642738422008,10.2334368540005,80.6));
#98395=CARTESIAN_POINT('Ctrl Pts',(115.669599337579,9.762546306575,80.2));
#98396=CARTESIAN_POINT('Ctrl Pts',(115.655894788818,10.0027965858745,80.4056749851139));
#98397=CARTESIAN_POINT('Ctrl Pts',(115.642738422008,10.2334368540005,80.6));
#98398=CARTESIAN_POINT('',(116.082281466203,10.0623774235676,80.2));
#98399=CARTESIAN_POINT('Ctrl Pts',(115.642738422008,10.2334368540005,80.6));
#98400=CARTESIAN_POINT('Ctrl Pts',(115.858024811002,10.1496526431759,80.4056749851125));
#98401=CARTESIAN_POINT('Ctrl Pts',(116.082281466203,10.0623774235676,80.2));
#98402=CARTESIAN_POINT('',(116.888418823398,10.7508837701784,80.2));
#98403=CARTESIAN_POINT('Origin',(110.,18.,80.2));
#98404=CARTESIAN_POINT('',(116.788225099391,11.2117749006091,80.6));
#98405=CARTESIAN_POINT('Ctrl Pts',(116.888418823398,10.7508837701784,80.2));
#98406=CARTESIAN_POINT('Ctrl Pts',(116.837299576455,10.9860323061133,80.4056749851139));
#98407=CARTESIAN_POINT('Ctrl Pts',(116.788225099391,11.2117749006091,80.6));
#98408=CARTESIAN_POINT('',(117.249116229822,11.1115811766025,80.2));
#98409=CARTESIAN_POINT('Ctrl Pts',(116.788225099391,11.2117749006091,80.6));
#98410=CARTESIAN_POINT('Ctrl Pts',(117.013967693888,11.1627004235446,80.405674985113));
#98411=CARTESIAN_POINT('Ctrl Pts',(117.249116229822,11.1115811766025,80.2));
#98412=CARTESIAN_POINT('',(117.937622576432,11.9177185337975,80.2));
#98413=CARTESIAN_POINT('Origin',(110.,18.,80.2));
#98414=CARTESIAN_POINT('',(117.766563145999,12.3572615779923,80.6));
#98415=CARTESIAN_POINT('Ctrl Pts',(117.937622576432,11.9177185337975,80.2));
#98416=CARTESIAN_POINT('Ctrl Pts',(117.850347356824,12.141975188999,80.4056749851133));
#98417=CARTESIAN_POINT('Ctrl Pts',(117.766563145999,12.3572615779923,80.6));
#98418=CARTESIAN_POINT('',(118.237453693425,12.3304006624208,80.2));
#98419=CARTESIAN_POINT('Ctrl Pts',(117.766563145999,12.3572615779923,80.6));
#98420=CARTESIAN_POINT('Ctrl Pts',(117.997203414126,12.3441052111817,80.4056749851134));
#98421=CARTESIAN_POINT('Ctrl Pts',(118.237453693425,12.3304006624208,80.2));
#98422=CARTESIAN_POINT('',(118.791375718177,13.2343192530493,80.2));
#98423=CARTESIAN_POINT('Origin',(110.,18.,80.2));
#98424=CARTESIAN_POINT('',(118.553662632208,13.6416912025004,80.6));
#98425=CARTESIAN_POINT('Ctrl Pts',(118.791375718177,13.2343192530493,80.2));
#98426=CARTESIAN_POINT('Ctrl Pts',(118.670093531458,13.4421620844014,80.4056749851128));
#98427=CARTESIAN_POINT('Ctrl Pts',(118.553662632208,13.6416912025004,80.6));
#98428=CARTESIAN_POINT('Ctrl Pts',(118.553662632208,13.6416912025004,80.6));
#98429=CARTESIAN_POINT('Ctrl Pts',(118.783521445112,13.6647768993581,80.4056749851135));
#98430=CARTESIAN_POINT('Ctrl Pts',(119.022957708555,13.6888245002517,80.2));
#98431=CARTESIAN_POINT('',(119.6,18.,80.6));
#98432=CARTESIAN_POINT('Ctrl Pts',(119.996746905394,17.7449484179612,80.2));
#98433=CARTESIAN_POINT('Ctrl Pts',(119.794325014887,17.8750767761442,80.4056749851131));
#98434=CARTESIAN_POINT('Ctrl Pts',(119.6,18.,80.6));
#98435=CARTESIAN_POINT('',(119.996746905394,18.2550515820388,80.2));
#98436=CARTESIAN_POINT('Ctrl Pts',(119.6,18.,80.6));
#98437=CARTESIAN_POINT('Ctrl Pts',(119.794325014887,18.124923223856,80.4056749851128));
#98438=CARTESIAN_POINT('Ctrl Pts',(119.996746905394,18.2550515820388,80.2));
#98439=CARTESIAN_POINT('',(119.913569220132,19.3119242804578,80.2));
#98440=CARTESIAN_POINT('Origin',(110.,18.,80.2));
#98441=CARTESIAN_POINT('',(119.481808069713,19.5017708643862,80.6));
#98442=CARTESIAN_POINT('Ctrl Pts',(119.913569220132,19.3119242804577,80.2));
#98443=CARTESIAN_POINT('Ctrl Pts',(119.693282918898,19.4087847824621,80.4056749851132));
#98444=CARTESIAN_POINT('Ctrl Pts',(119.481808069713,19.5017708643862,80.6));
#98445=CARTESIAN_POINT('',(119.833771504544,19.815747228118,80.2));
#98446=CARTESIAN_POINT('Ctrl Pts',(119.481808069713,19.5017708643862,80.6));
#98447=CARTESIAN_POINT('Ctrl Pts',(119.654198323507,19.655555205805,80.4056749851143));
#98448=CARTESIAN_POINT('Ctrl Pts',(119.833771504544,19.815747228118,80.2));
#98449=CARTESIAN_POINT('',(119.58628655942,20.8465962131424,80.2));
#98450=CARTESIAN_POINT('Origin',(110.,18.,80.2));
#98451=CARTESIAN_POINT('',(119.130142556433,20.9665631459995,80.6));
#98452=CARTESIAN_POINT('Ctrl Pts',(119.58628655942,20.8465962131424,80.2));
#98453=CARTESIAN_POINT('Ctrl Pts',(119.353560027284,20.907803831947,80.4056749851133));
#98454=CARTESIAN_POINT('Ctrl Pts',(119.130142556433,20.9665631459995,80.6));
#98455=CARTESIAN_POINT('',(119.428656012836,21.3317331513213,80.2));
#98456=CARTESIAN_POINT('Ctrl Pts',(119.130142556433,20.9665631459995,80.6));
#98457=CARTESIAN_POINT('Ctrl Pts',(119.276353228957,21.1454219241167,80.4056749851128));
#98458=CARTESIAN_POINT('Ctrl Pts',(119.428656012836,21.3317331513213,80.2));
#98459=CARTESIAN_POINT('',(119.022957708555,22.3111754997483,80.2));
#98460=CARTESIAN_POINT('Origin',(110.,18.,80.2));
#98461=CARTESIAN_POINT('',(118.553662632208,22.3583087974996,80.6));
#98462=CARTESIAN_POINT('Ctrl Pts',(119.022957708555,22.3111754997483,80.2));
#98463=CARTESIAN_POINT('Ctrl Pts',(118.783521445111,22.335223100642,80.4056749851144));
#98464=CARTESIAN_POINT('Ctrl Pts',(118.553662632208,22.3583087974996,80.6));
#98465=CARTESIAN_POINT('',(118.791375718177,22.7656807469507,80.2));
#98466=CARTESIAN_POINT('Ctrl Pts',(118.553662632208,22.3583087974996,80.6));
#98467=CARTESIAN_POINT('Ctrl Pts',(118.670093531459,22.5578379155991,80.4056749851123));
#98468=CARTESIAN_POINT('Ctrl Pts',(118.791375718177,22.7656807469507,80.2));
#98469=CARTESIAN_POINT('',(118.237453693425,23.6695993375792,80.2));
#98470=CARTESIAN_POINT('Origin',(110.,18.,80.2));
#98471=CARTESIAN_POINT('',(117.766563145999,23.6427384220077,80.6));
#98472=CARTESIAN_POINT('Ctrl Pts',(118.237453693425,23.6695993375792,80.2));
#98473=CARTESIAN_POINT('Ctrl Pts',(117.997203414127,23.6558947888183,80.4056749851127));
#98474=CARTESIAN_POINT('Ctrl Pts',(117.766563145999,23.6427384220077,80.6));
#98475=CARTESIAN_POINT('',(117.937622576432,24.0822814662025,80.2));
#98476=CARTESIAN_POINT('Ctrl Pts',(117.766563145999,23.6427384220077,80.6));
#98477=CARTESIAN_POINT('Ctrl Pts',(117.850347356824,23.8580248110013,80.4056749851131));
#98478=CARTESIAN_POINT('Ctrl Pts',(117.937622576432,24.0822814662025,80.2));
#98479=CARTESIAN_POINT('',(117.249116229822,24.8884188233975,80.2));
#98480=CARTESIAN_POINT('Origin',(110.,18.,80.2));
#98481=CARTESIAN_POINT('',(116.788225099391,24.7882250993908,80.6));
#98482=CARTESIAN_POINT('Ctrl Pts',(117.249116229822,24.8884188233975,80.2));
#98483=CARTESIAN_POINT('Ctrl Pts',(117.013967693888,24.8372995764555,80.4056749851127));
#98484=CARTESIAN_POINT('Ctrl Pts',(116.788225099391,24.7882250993908,80.6));
#98485=CARTESIAN_POINT('',(116.888418823398,25.2491162298216,80.2));
#98486=CARTESIAN_POINT('Ctrl Pts',(116.788225099391,24.7882250993908,80.6));
#98487=CARTESIAN_POINT('Ctrl Pts',(116.837299576455,25.0139676938872,80.4056749851135));
#98488=CARTESIAN_POINT('Ctrl Pts',(116.888418823398,25.2491162298216,80.2));
#98489=CARTESIAN_POINT('',(116.082281466203,25.9376225764324,80.2));
#98490=CARTESIAN_POINT('Origin',(110.,18.,80.2));
#98491=CARTESIAN_POINT('',(115.642738422008,25.7665631459995,80.6));
#98492=CARTESIAN_POINT('Ctrl Pts',(116.082281466202,25.9376225764324,80.2));
#98493=CARTESIAN_POINT('Ctrl Pts',(115.858024811001,25.8503473568238,80.4056749851132));
#98494=CARTESIAN_POINT('Ctrl Pts',(115.642738422008,25.7665631459995,80.6));
#98495=CARTESIAN_POINT('',(115.669599337579,26.237453693425,80.2));
#98496=CARTESIAN_POINT('Ctrl Pts',(115.642738422008,25.7665631459995,80.6));
#98497=CARTESIAN_POINT('Ctrl Pts',(115.655894788818,25.9972034141258,80.4056749851137));
#98498=CARTESIAN_POINT('Ctrl Pts',(115.669599337579,26.237453693425,80.2));
#98499=CARTESIAN_POINT('',(114.765680746951,26.7913757181765,80.2));
#98500=CARTESIAN_POINT('Origin',(110.,18.,80.2));
#98501=CARTESIAN_POINT('',(114.3583087975,26.5536626322083,80.6));
#98502=CARTESIAN_POINT('Ctrl Pts',(114.765680746951,26.7913757181765,80.2));
#98503=CARTESIAN_POINT('Ctrl Pts',(114.557837915598,26.670093531458,80.4056749851134));
#98504=CARTESIAN_POINT('Ctrl Pts',(114.3583087975,26.5536626322083,80.6));
#98505=CARTESIAN_POINT('',(114.311175499748,27.0229577085549,80.2));
#98506=CARTESIAN_POINT('Ctrl Pts',(114.3583087975,26.5536626322083,80.6));
#98507=CARTESIAN_POINT('Ctrl Pts',(114.335223100642,26.783521445112,80.4056749851139));
#98508=CARTESIAN_POINT('Ctrl Pts',(114.311175499748,27.0229577085549,80.2));
#98509=CARTESIAN_POINT('',(113.331733151321,27.4286560128359,80.2));
#98510=CARTESIAN_POINT('Origin',(110.,18.,80.2));
#98511=CARTESIAN_POINT('',(112.966563146,27.1301425564335,80.6));
#98512=CARTESIAN_POINT('Ctrl Pts',(113.331733151321,27.4286560128359,80.2));
#98513=CARTESIAN_POINT('Ctrl Pts',(113.145421924116,27.276353228957,80.4056749851134));
#98514=CARTESIAN_POINT('Ctrl Pts',(112.966563146,27.1301425564335,80.6));
#98515=CARTESIAN_POINT('',(112.846596213142,27.5862865594204,80.2));
#98516=CARTESIAN_POINT('Ctrl Pts',(112.966563146,27.1301425564335,80.6));
#98517=CARTESIAN_POINT('Ctrl Pts',(112.907803831947,27.3535600272837,80.4056749851137));
#98518=CARTESIAN_POINT('Ctrl Pts',(112.846596213142,27.5862865594204,80.2));
#98519=CARTESIAN_POINT('',(111.815747228118,27.833771504544,80.2));
#98520=CARTESIAN_POINT('Origin',(110.,18.,80.2));
#98521=CARTESIAN_POINT('',(111.501770864386,27.4818080697133,80.6));
#98522=CARTESIAN_POINT('Ctrl Pts',(111.815747228118,27.833771504544,80.2));
#98523=CARTESIAN_POINT('Ctrl Pts',(111.655555205806,27.6541983235079,80.4056749851134));
#98524=CARTESIAN_POINT('Ctrl Pts',(111.501770864386,27.4818080697133,80.6));
#98525=CARTESIAN_POINT('',(111.311924280458,27.9135692201318,80.2));
#98526=CARTESIAN_POINT('Ctrl Pts',(111.501770864386,27.4818080697133,80.6));
#98527=CARTESIAN_POINT('Ctrl Pts',(111.408784782462,27.6932829188972,80.4056749851139));
#98528=CARTESIAN_POINT('Ctrl Pts',(111.311924280458,27.9135692201318,80.2));
#98529=CARTESIAN_POINT('',(110.255051582039,27.9967469053937,80.2));
#98530=CARTESIAN_POINT('Origin',(110.,18.,80.2));
#98531=CARTESIAN_POINT('',(110.,27.6,80.6));
#98532=CARTESIAN_POINT('Ctrl Pts',(110.255051582039,27.9967469053937,80.2));
#98533=CARTESIAN_POINT('Ctrl Pts',(110.124923223856,27.7943250148868,80.4056749851132));
#98534=CARTESIAN_POINT('Ctrl Pts',(110.,27.6,80.6));
#98535=CARTESIAN_POINT('',(109.744948417961,27.9967469053937,80.2));
#98536=CARTESIAN_POINT('Ctrl Pts',(110.,27.6,80.6));
#98537=CARTESIAN_POINT('Ctrl Pts',(109.875076776144,27.7943250148865,80.4056749851135));
#98538=CARTESIAN_POINT('Ctrl Pts',(109.744948417961,27.9967469053938,80.2));
#98539=CARTESIAN_POINT('',(108.688075719542,27.9135692201318,80.2));
#98540=CARTESIAN_POINT('Origin',(110.,18.,80.2));
#98541=CARTESIAN_POINT('',(108.498229135614,27.4818080697133,80.6));
#98542=CARTESIAN_POINT('Ctrl Pts',(108.688075719542,27.9135692201318,80.2));
#98543=CARTESIAN_POINT('Ctrl Pts',(108.591215217538,27.693282918897,80.4056749851141));
#98544=CARTESIAN_POINT('Ctrl Pts',(108.498229135614,27.4818080697133,80.6));
#98545=CARTESIAN_POINT('',(108.184252771882,27.833771504544,80.2));
#98546=CARTESIAN_POINT('Ctrl Pts',(108.498229135614,27.4818080697133,80.6));
#98547=CARTESIAN_POINT('Ctrl Pts',(108.344444794194,27.6541983235076,80.4056749851136));
#98548=CARTESIAN_POINT('Ctrl Pts',(108.184252771882,27.833771504544,80.2));
#98549=CARTESIAN_POINT('',(107.153403786858,27.5862865594204,80.2));
#98550=CARTESIAN_POINT('Origin',(110.,18.,80.2));
#98551=CARTESIAN_POINT('',(107.033436854,27.1301425564335,80.6));
#98552=CARTESIAN_POINT('Ctrl Pts',(107.153403786858,27.5862865594204,80.2));
#98553=CARTESIAN_POINT('Ctrl Pts',(107.092196168053,27.3535600272838,80.4056749851136));
#98554=CARTESIAN_POINT('Ctrl Pts',(107.033436854,27.1301425564335,80.6));
#98555=CARTESIAN_POINT('',(106.668266848679,27.4286560128359,80.2));
#98556=CARTESIAN_POINT('Ctrl Pts',(107.033436854,27.1301425564335,80.6));
#98557=CARTESIAN_POINT('Ctrl Pts',(106.854578075884,27.276353228957,80.4056749851134));
#98558=CARTESIAN_POINT('Ctrl Pts',(106.668266848679,27.4286560128359,80.2));
#98559=CARTESIAN_POINT('',(105.688824500252,27.0229577085549,80.2));
#98560=CARTESIAN_POINT('Origin',(110.,18.,80.2));
#98561=CARTESIAN_POINT('',(105.6416912025,26.5536626322083,80.6));
#98562=CARTESIAN_POINT('Ctrl Pts',(105.688824500252,27.0229577085549,80.2));
#98563=CARTESIAN_POINT('Ctrl Pts',(105.664776899358,26.7835214451122,80.4056749851137));
#98564=CARTESIAN_POINT('Ctrl Pts',(105.6416912025,26.5536626322083,80.6));
#98565=CARTESIAN_POINT('',(105.234319253049,26.7913757181765,80.2));
#98566=CARTESIAN_POINT('Ctrl Pts',(105.6416912025,26.5536626322083,80.6));
#98567=CARTESIAN_POINT('Ctrl Pts',(105.442162084403,26.6700935314577,80.4056749851139));
#98568=CARTESIAN_POINT('Ctrl Pts',(105.234319253049,26.7913757181765,80.2));
#98569=CARTESIAN_POINT('',(104.330400662421,26.237453693425,80.2));
#98570=CARTESIAN_POINT('Origin',(110.,18.,80.2));
#98571=CARTESIAN_POINT('',(104.357261577992,25.7665631459995,80.6));
#98572=CARTESIAN_POINT('Ctrl Pts',(104.330400662421,26.237453693425,80.2));
#98573=CARTESIAN_POINT('Ctrl Pts',(104.344105211182,25.9972034141259,80.4056749851136));
#98574=CARTESIAN_POINT('Ctrl Pts',(104.357261577992,25.7665631459995,80.6));
#98575=CARTESIAN_POINT('',(103.917718533797,25.9376225764324,80.2));
#98576=CARTESIAN_POINT('Ctrl Pts',(104.357261577992,25.7665631459995,80.6));
#98577=CARTESIAN_POINT('Ctrl Pts',(104.141975188998,25.8503473568243,80.4056749851121));
#98578=CARTESIAN_POINT('Ctrl Pts',(103.917718533797,25.9376225764324,80.2));
#98579=CARTESIAN_POINT('',(103.111581176602,25.2491162298216,80.2));
#98580=CARTESIAN_POINT('Origin',(110.,18.,80.2));
#98581=CARTESIAN_POINT('',(103.211774900609,24.7882250993908,80.6));
#98582=CARTESIAN_POINT('Ctrl Pts',(103.111581176602,25.2491162298216,80.2));
#98583=CARTESIAN_POINT('Ctrl Pts',(103.162700423545,25.013967693886,80.4056749851146));
#98584=CARTESIAN_POINT('Ctrl Pts',(103.211774900609,24.7882250993908,80.6));
#98585=CARTESIAN_POINT('',(102.750883770178,24.8884188233975,80.2));
#98586=CARTESIAN_POINT('Ctrl Pts',(103.211774900609,24.7882250993908,80.6));
#98587=CARTESIAN_POINT('Ctrl Pts',(102.986032306113,24.8372995764552,80.4056749851138));
#98588=CARTESIAN_POINT('Ctrl Pts',(102.750883770178,24.8884188233975,80.2));
#98589=CARTESIAN_POINT('',(102.062377423568,24.0822814662025,80.2));
#98590=CARTESIAN_POINT('Origin',(110.,18.,80.2));
#98591=CARTESIAN_POINT('',(102.233436854001,23.6427384220077,80.6));
#98592=CARTESIAN_POINT('Ctrl Pts',(102.062377423568,24.0822814662025,80.2));
#98593=CARTESIAN_POINT('Ctrl Pts',(102.149652643176,23.8580248110016,80.4056749851128));
#98594=CARTESIAN_POINT('Ctrl Pts',(102.233436854001,23.6427384220077,80.6));
#98595=CARTESIAN_POINT('',(101.762546306575,23.6695993375792,80.2));
#98596=CARTESIAN_POINT('Ctrl Pts',(102.233436854001,23.6427384220077,80.6));
#98597=CARTESIAN_POINT('Ctrl Pts',(102.002796585873,23.6558947888183,80.4056749851127));
#98598=CARTESIAN_POINT('Ctrl Pts',(101.762546306575,23.6695993375792,80.2));
#98599=CARTESIAN_POINT('',(101.208624281823,22.7656807469507,80.2));
#98600=CARTESIAN_POINT('Origin',(110.,18.,80.2));
#98601=CARTESIAN_POINT('',(101.446337367792,22.3583087974996,80.6));
#98602=CARTESIAN_POINT('Ctrl Pts',(101.208624281823,22.7656807469507,80.2));
#98603=CARTESIAN_POINT('Ctrl Pts',(101.329906468542,22.5578379155986,80.4056749851127));
#98604=CARTESIAN_POINT('Ctrl Pts',(101.446337367792,22.3583087974996,80.6));
#98605=CARTESIAN_POINT('',(100.977042291445,22.3111754997483,80.2));
#98606=CARTESIAN_POINT('Ctrl Pts',(101.446337367792,22.3583087974996,80.6));
#98607=CARTESIAN_POINT('Ctrl Pts',(101.216478554888,22.3352231006419,80.405674985114));
#98608=CARTESIAN_POINT('Ctrl Pts',(100.977042291445,22.3111754997483,80.2));
#98609=CARTESIAN_POINT('',(100.571343987164,21.3317331513213,80.2));
#98610=CARTESIAN_POINT('Origin',(110.,18.,80.2));
#98611=CARTESIAN_POINT('',(100.869857443567,20.9665631459995,80.6));
#98612=CARTESIAN_POINT('Ctrl Pts',(100.571343987164,21.3317331513213,80.2));
#98613=CARTESIAN_POINT('Ctrl Pts',(100.723646771043,21.145421924116,80.4056749851135));
#98614=CARTESIAN_POINT('Ctrl Pts',(100.869857443567,20.9665631459995,80.6));
#98615=CARTESIAN_POINT('',(100.41371344058,20.8465962131424,80.2));
#98616=CARTESIAN_POINT('Ctrl Pts',(100.869857443567,20.9665631459995,80.6));
#98617=CARTESIAN_POINT('Ctrl Pts',(100.646439972715,20.9078038319469,80.4056749851127));
#98618=CARTESIAN_POINT('Ctrl Pts',(100.41371344058,20.8465962131424,80.2));
#98619=CARTESIAN_POINT('',(100.166228495456,19.815747228118,80.2));
#98620=CARTESIAN_POINT('Origin',(110.,18.,80.2));
#98621=CARTESIAN_POINT('',(100.518191930287,19.5017708643862,80.6));
#98622=CARTESIAN_POINT('Ctrl Pts',(100.166228495456,19.815747228118,80.2));
#98623=CARTESIAN_POINT('Ctrl Pts',(100.345801676492,19.655555205806,80.4056749851131));
#98624=CARTESIAN_POINT('Ctrl Pts',(100.518191930287,19.5017708643862,80.6));
#98625=CARTESIAN_POINT('',(100.086430779868,19.3119242804578,80.2));
#98626=CARTESIAN_POINT('Ctrl Pts',(100.518191930287,19.5017708643862,80.6));
#98627=CARTESIAN_POINT('Ctrl Pts',(100.306717081102,19.4087847824621,80.4056749851134));
#98628=CARTESIAN_POINT('Ctrl Pts',(100.086430779868,19.3119242804578,80.2));
#98629=CARTESIAN_POINT('',(100.003253094606,18.2550515820388,80.2));
#98630=CARTESIAN_POINT('Origin',(110.,18.,80.2));
#98631=CARTESIAN_POINT('Ctrl Pts',(100.003253094606,18.2550515820388,80.2));
#98632=CARTESIAN_POINT('Ctrl Pts',(100.205674985113,18.1249232238562,80.4056749851126));
#98633=CARTESIAN_POINT('Ctrl Pts',(100.4,18.,80.6));
#98634=CARTESIAN_POINT('Origin',(118.553662632208,13.6416912025004,81.));
#98635=CARTESIAN_POINT('',(118.553662632208,13.6416912025004,81.));
#98636=CARTESIAN_POINT('Origin',(118.973071474257,12.9229449167979,81.));
#98637=CARTESIAN_POINT('',(118.791375718177,13.2343192530493,73.5));
#98638=CARTESIAN_POINT('Origin',(117.766563145999,12.3572615779923,81.));
#98639=CARTESIAN_POINT('',(117.766563145999,12.3572615779923,81.));
#98640=CARTESIAN_POINT('',(118.237453693425,12.3304006624208,73.5));
#98641=CARTESIAN_POINT('Origin',(118.06837167853,11.5817542539188,81.));
#98642=CARTESIAN_POINT('',(117.937622576432,11.9177185337975,73.5));
#98643=CARTESIAN_POINT('Origin',(110.,18.,73.5));
#98644=CARTESIAN_POINT('',(117.249116229822,11.1115811766025,73.5));
#98645=CARTESIAN_POINT('Origin',(110.,18.,73.5));
#98646=CARTESIAN_POINT('Origin',(116.965001794687,10.3986021022446,81.));
#98647=CARTESIAN_POINT('',(116.788225099391,11.2117749006091,81.));
#98648=CARTESIAN_POINT('',(116.888418823398,10.7508837701784,73.5));
#98649=CARTESIAN_POINT('Origin',(116.788225099391,11.2117749006091,81.));
#98650=CARTESIAN_POINT('Origin',(110.,18.,73.5));
#98651=CARTESIAN_POINT('',(116.082281466203,10.0623774235676,73.5));
#98652=CARTESIAN_POINT('Origin',(115.642738422008,10.2334368540005,81.));
#98653=CARTESIAN_POINT('',(115.642738422008,10.2334368540005,81.));
#98654=CARTESIAN_POINT('Origin',(115.690130451144,9.40262159440644,81.));
#98655=CARTESIAN_POINT('',(115.669599337579,9.762546306575,73.5));
#98656=CARTESIAN_POINT('Origin',(114.3583087975,9.44633736779169,81.));
#98657=CARTESIAN_POINT('',(114.3583087975,9.44633736779169,81.));
#98658=CARTESIAN_POINT('',(114.765680746951,9.20862428182348,73.5));
#98659=CARTESIAN_POINT('Origin',(114.275149211433,8.61833707597702,81.));
#98660=CARTESIAN_POINT('',(114.311175499748,8.97704229144512,73.5));
#98661=CARTESIAN_POINT('Origin',(110.,18.,73.5));
#98662=CARTESIAN_POINT('',(113.331733151321,8.57134398716408,73.5));
#98663=CARTESIAN_POINT('Origin',(110.,18.,73.5));
#98664=CARTESIAN_POINT('Origin',(112.754899609729,8.06506023469121,81.));
#98665=CARTESIAN_POINT('',(112.966563146,8.86985744356654,81.));
#98666=CARTESIAN_POINT('',(112.846596213142,8.41371344057965,73.5));
#98667=CARTESIAN_POINT('Origin',(112.966563146,8.86985744356654,81.));
#98668=CARTESIAN_POINT('Origin',(110.,18.,73.5));
#98669=CARTESIAN_POINT('',(111.815747228118,8.16622849545598,73.5));
#98670=CARTESIAN_POINT('Origin',(111.501770864386,8.51819193028669,81.));
#98671=CARTESIAN_POINT('',(111.501770864386,8.51819193028669,81.));
#98672=CARTESIAN_POINT('Origin',(111.166815236647,7.75641458260198,81.));
#98673=CARTESIAN_POINT('',(111.311924280458,8.08643077986816,73.5));
#98674=CARTESIAN_POINT('Origin',(110.,8.40000000000002,81.));
#98675=CARTESIAN_POINT('',(110.,8.40000000000002,81.));
#98676=CARTESIAN_POINT('',(110.255051582039,8.00325309460625,73.5));
#98677=CARTESIAN_POINT('Origin',(109.55,7.70000000000001,81.));
#98678=CARTESIAN_POINT('',(109.744948417961,8.00325309460625,73.5));
#98679=CARTESIAN_POINT('Origin',(110.,18.,73.5));
#98680=CARTESIAN_POINT('',(108.688075719542,8.08643077986816,73.5));
#98681=CARTESIAN_POINT('Origin',(110.,18.,73.5));
#98682=CARTESIAN_POINT('Origin',(107.944265256818,7.89720560113819,81.));
#98683=CARTESIAN_POINT('',(108.498229135614,8.51819193028669,81.));
#98684=CARTESIAN_POINT('',(108.184252771882,8.16622849545598,73.5));
#98685=CARTESIAN_POINT('Origin',(108.498229135614,8.51819193028669,81.));
#98686=CARTESIAN_POINT('Origin',(110.,18.,73.5));
#98687=CARTESIAN_POINT('',(107.153403786858,8.41371344057964,73.5));
#98688=CARTESIAN_POINT('Origin',(107.033436854001,8.86985744356654,81.));
#98689=CARTESIAN_POINT('',(107.033436854001,8.86985744356654,81.));
#98690=CARTESIAN_POINT('Origin',(106.389149525605,8.34317552962865,81.));
#98691=CARTESIAN_POINT('',(106.668266848679,8.57134398716408,73.5));
#98692=CARTESIAN_POINT('Origin',(105.6416912025,9.44633736779169,81.));
#98693=CARTESIAN_POINT('',(105.6416912025,9.44633736779169,81.));
#98694=CARTESIAN_POINT('',(105.688824500252,8.97704229144512,73.5));
#98695=CARTESIAN_POINT('Origin',(104.922944916798,9.02692852574262,81.));
#98696=CARTESIAN_POINT('',(105.234319253049,9.20862428182348,73.5));
#98697=CARTESIAN_POINT('Origin',(110.,18.,73.5));
#98698=CARTESIAN_POINT('',(104.330400662421,9.76254630657499,73.5));
#98699=CARTESIAN_POINT('Origin',(110.,18.,73.5));
#98700=CARTESIAN_POINT('Origin',(103.581754253919,9.93162832146966,81.));
#98701=CARTESIAN_POINT('',(104.357261577992,10.2334368540005,81.));
#98702=CARTESIAN_POINT('',(103.917718533797,10.0623774235676,73.5));
#98703=CARTESIAN_POINT('Origin',(104.357261577992,10.2334368540005,81.));
#98704=CARTESIAN_POINT('Origin',(110.,18.,73.5));
#98705=CARTESIAN_POINT('',(103.111581176602,10.7508837701784,73.5));
#98706=CARTESIAN_POINT('Origin',(103.211774900609,11.2117749006092,81.));
#98707=CARTESIAN_POINT('',(103.211774900609,11.2117749006092,81.));
#98708=CARTESIAN_POINT('Origin',(102.398602102245,11.0349982053125,81.));
#98709=CARTESIAN_POINT('',(102.750883770178,11.1115811766025,73.5));
#98710=CARTESIAN_POINT('Origin',(102.233436854001,12.3572615779923,81.));
#98711=CARTESIAN_POINT('',(102.233436854001,12.3572615779923,81.));
#98712=CARTESIAN_POINT('',(102.062377423568,11.9177185337975,73.5));
#98713=CARTESIAN_POINT('Origin',(101.402621594406,12.3098695488563,81.));
#98714=CARTESIAN_POINT('',(101.762546306575,12.3304006624208,73.5));
#98715=CARTESIAN_POINT('Origin',(110.,18.,73.5));
#98716=CARTESIAN_POINT('',(101.208624281823,13.2343192530494,73.5));
#98717=CARTESIAN_POINT('Origin',(110.,18.,73.5));
#98718=CARTESIAN_POINT('Origin',(100.618337075977,13.7248507885675,81.));
#98719=CARTESIAN_POINT('',(101.446337367792,13.6416912025004,81.));
#98720=CARTESIAN_POINT('',(100.977042291445,13.6888245002517,73.5));
#98721=CARTESIAN_POINT('Origin',(101.446337367792,13.6416912025004,81.));
#98722=CARTESIAN_POINT('Origin',(110.,18.,73.5));
#98723=CARTESIAN_POINT('',(100.571343987164,14.6682668486788,73.5));
#98724=CARTESIAN_POINT('Origin',(100.869857443567,15.0334368540005,81.));
#98725=CARTESIAN_POINT('',(100.869857443567,15.0334368540005,81.));
#98726=CARTESIAN_POINT('Origin',(100.065060234691,15.2451003902709,81.));
#98727=CARTESIAN_POINT('',(100.41371344058,15.1534037868576,73.5));
#98728=CARTESIAN_POINT('Origin',(100.518191930287,16.4982291356138,81.));
#98729=CARTESIAN_POINT('',(100.518191930287,16.4982291356138,81.));
#98730=CARTESIAN_POINT('',(100.166228495456,16.184252771882,73.5));
#98731=CARTESIAN_POINT('Origin',(99.756414582602,16.8331847633534,81.));
#98732=CARTESIAN_POINT('',(100.086430779868,16.6880757195422,73.5));
#98733=CARTESIAN_POINT('Origin',(110.,18.,73.5));
#98734=CARTESIAN_POINT('',(100.003253094606,17.7449484179612,73.5));
#98735=CARTESIAN_POINT('Origin',(110.,18.,73.5));
#98736=CARTESIAN_POINT('Origin',(99.7,18.45,81.));
#98737=CARTESIAN_POINT('',(100.4,18.,81.));
#98738=CARTESIAN_POINT('',(100.003253094606,18.2550515820388,73.5));
#98739=CARTESIAN_POINT('Origin',(100.4,18.,81.));
#98740=CARTESIAN_POINT('Origin',(110.,18.,73.5));
#98741=CARTESIAN_POINT('',(100.086430779868,19.3119242804578,73.5));
#98742=CARTESIAN_POINT('Origin',(100.518191930287,19.5017708643862,81.));
#98743=CARTESIAN_POINT('',(100.518191930287,19.5017708643862,81.));
#98744=CARTESIAN_POINT('Origin',(99.8972056011382,20.0557347431822,81.));
#98745=CARTESIAN_POINT('',(100.166228495456,19.815747228118,73.5));
#98746=CARTESIAN_POINT('Origin',(100.869857443567,20.9665631459995,81.));
#98747=CARTESIAN_POINT('',(100.869857443567,20.9665631459995,81.));
#98748=CARTESIAN_POINT('',(100.41371344058,20.8465962131424,73.5));
#98749=CARTESIAN_POINT('Origin',(100.343175529629,21.6108504743948,81.));
#98750=CARTESIAN_POINT('',(100.571343987164,21.3317331513213,73.5));
#98751=CARTESIAN_POINT('Origin',(110.,18.,73.5));
#98752=CARTESIAN_POINT('',(100.977042291445,22.3111754997483,73.5));
#98753=CARTESIAN_POINT('Origin',(110.,18.,73.5));
#98754=CARTESIAN_POINT('Origin',(101.026928525743,23.0770550832021,81.));
#98755=CARTESIAN_POINT('',(101.446337367792,22.3583087974996,81.));
#98756=CARTESIAN_POINT('',(101.208624281823,22.7656807469507,73.5));
#98757=CARTESIAN_POINT('Origin',(101.446337367792,22.3583087974996,81.));
#98758=CARTESIAN_POINT('Origin',(110.,18.,73.5));
#98759=CARTESIAN_POINT('',(101.762546306575,23.6695993375792,73.5));
#98760=CARTESIAN_POINT('Origin',(102.233436854001,23.6427384220077,81.));
#98761=CARTESIAN_POINT('',(102.233436854001,23.6427384220077,81.));
#98762=CARTESIAN_POINT('Origin',(101.93162832147,24.4182457460812,81.));
#98763=CARTESIAN_POINT('',(102.062377423568,24.0822814662025,73.5));
#98764=CARTESIAN_POINT('Origin',(103.211774900609,24.7882250993908,81.));
#98765=CARTESIAN_POINT('',(103.211774900609,24.7882250993908,81.));
#98766=CARTESIAN_POINT('',(102.750883770178,24.8884188233975,73.5));
#98767=CARTESIAN_POINT('Origin',(103.034998205313,25.6013978977554,81.));
#98768=CARTESIAN_POINT('',(103.111581176602,25.2491162298216,73.5));
#98769=CARTESIAN_POINT('Origin',(110.,18.,73.5));
#98770=CARTESIAN_POINT('',(103.917718533797,25.9376225764324,73.5));
#98771=CARTESIAN_POINT('Origin',(110.,18.,73.5));
#98772=CARTESIAN_POINT('Origin',(104.309869548856,26.5973784055936,81.));
#98773=CARTESIAN_POINT('',(104.357261577992,25.7665631459995,81.));
#98774=CARTESIAN_POINT('',(104.330400662421,26.237453693425,73.5));
#98775=CARTESIAN_POINT('Origin',(104.357261577992,25.7665631459995,81.));
#98776=CARTESIAN_POINT('Origin',(110.,18.,73.5));
#98777=CARTESIAN_POINT('',(105.234319253049,26.7913757181765,73.5));
#98778=CARTESIAN_POINT('Origin',(105.6416912025,26.5536626322083,81.));
#98779=CARTESIAN_POINT('',(105.6416912025,26.5536626322083,81.));
#98780=CARTESIAN_POINT('Origin',(105.724850788567,27.381662924023,81.));
#98781=CARTESIAN_POINT('',(105.688824500252,27.0229577085549,73.5));
#98782=CARTESIAN_POINT('Origin',(107.033436854,27.1301425564335,81.));
#98783=CARTESIAN_POINT('',(107.033436854,27.1301425564335,81.));
#98784=CARTESIAN_POINT('',(106.668266848679,27.4286560128359,73.5));
#98785=CARTESIAN_POINT('Origin',(107.245100390271,27.9349397653088,81.));
#98786=CARTESIAN_POINT('',(107.153403786858,27.5862865594204,73.5));
#98787=CARTESIAN_POINT('Origin',(110.,18.,73.5));
#98788=CARTESIAN_POINT('',(108.184252771882,27.833771504544,73.5));
#98789=CARTESIAN_POINT('Origin',(110.,18.,73.5));
#98790=CARTESIAN_POINT('Origin',(108.833184763353,28.243585417398,81.));
#98791=CARTESIAN_POINT('',(108.498229135614,27.4818080697133,81.));
#98792=CARTESIAN_POINT('',(108.688075719542,27.9135692201318,73.5));
#98793=CARTESIAN_POINT('Origin',(108.498229135614,27.4818080697133,81.));
#98794=CARTESIAN_POINT('Origin',(110.,18.,73.5));
#98795=CARTESIAN_POINT('',(109.744948417961,27.9967469053937,73.5));
#98796=CARTESIAN_POINT('Origin',(110.,27.6,81.));
#98797=CARTESIAN_POINT('',(110.,27.6,81.));
#98798=CARTESIAN_POINT('Origin',(110.45,28.3,81.));
#98799=CARTESIAN_POINT('',(110.255051582039,27.9967469053937,73.5));
#98800=CARTESIAN_POINT('Origin',(111.501770864386,27.4818080697133,81.));
#98801=CARTESIAN_POINT('',(111.501770864386,27.4818080697133,81.));
#98802=CARTESIAN_POINT('',(111.311924280458,27.9135692201318,73.5));
#98803=CARTESIAN_POINT('Origin',(112.055734743182,28.1027943988618,81.));
#98804=CARTESIAN_POINT('',(111.815747228118,27.833771504544,73.5));
#98805=CARTESIAN_POINT('Origin',(110.,18.,73.5));
#98806=CARTESIAN_POINT('',(112.846596213142,27.5862865594204,73.5));
#98807=CARTESIAN_POINT('Origin',(110.,18.,73.5));
#98808=CARTESIAN_POINT('Origin',(113.610850474395,27.6568244703713,81.));
#98809=CARTESIAN_POINT('',(112.966563146,27.1301425564335,81.));
#98810=CARTESIAN_POINT('',(113.331733151321,27.4286560128359,73.5));
#98811=CARTESIAN_POINT('Origin',(112.966563146,27.1301425564335,81.));
#98812=CARTESIAN_POINT('Origin',(110.,18.,73.5));
#98813=CARTESIAN_POINT('',(114.311175499748,27.0229577085549,73.5));
#98814=CARTESIAN_POINT('Origin',(114.3583087975,26.5536626322083,81.));
#98815=CARTESIAN_POINT('',(114.3583087975,26.5536626322083,81.));
#98816=CARTESIAN_POINT('Origin',(115.077055083202,26.9730714742574,81.));
#98817=CARTESIAN_POINT('',(114.765680746951,26.7913757181765,73.5));
#98818=CARTESIAN_POINT('Origin',(115.642738422008,25.7665631459995,81.));
#98819=CARTESIAN_POINT('',(115.642738422008,25.7665631459995,81.));
#98820=CARTESIAN_POINT('',(115.669599337579,26.237453693425,73.5));
#98821=CARTESIAN_POINT('Origin',(116.418245746081,26.0683716785304,81.));
#98822=CARTESIAN_POINT('',(116.082281466203,25.9376225764324,73.5));
#98823=CARTESIAN_POINT('Origin',(110.,18.,73.5));
#98824=CARTESIAN_POINT('',(116.888418823398,25.2491162298216,73.5));
#98825=CARTESIAN_POINT('Origin',(110.,18.,73.5));
#98826=CARTESIAN_POINT('Origin',(117.601397897755,24.9650017946875,81.));
#98827=CARTESIAN_POINT('',(116.788225099391,24.7882250993908,81.));
#98828=CARTESIAN_POINT('',(117.249116229822,24.8884188233975,73.5));
#98829=CARTESIAN_POINT('Origin',(116.788225099391,24.7882250993908,81.));
#98830=CARTESIAN_POINT('Origin',(110.,18.,73.5));
#98831=CARTESIAN_POINT('',(117.937622576432,24.0822814662025,73.5));
#98832=CARTESIAN_POINT('Origin',(117.766563145999,23.6427384220077,81.));
#98833=CARTESIAN_POINT('',(117.766563145999,23.6427384220077,81.));
#98834=CARTESIAN_POINT('Origin',(118.597378405594,23.6901304511437,81.));
#98835=CARTESIAN_POINT('',(118.237453693425,23.6695993375792,73.5));
#98836=CARTESIAN_POINT('Origin',(118.553662632208,22.3583087974996,81.));
#98837=CARTESIAN_POINT('',(118.553662632208,22.3583087974996,81.));
#98838=CARTESIAN_POINT('',(118.791375718177,22.7656807469507,73.5));
#98839=CARTESIAN_POINT('Origin',(119.381662924023,22.2751492114326,81.));
#98840=CARTESIAN_POINT('',(119.022957708555,22.3111754997483,73.5));
#98841=CARTESIAN_POINT('Origin',(110.,18.,73.5));
#98842=CARTESIAN_POINT('',(119.428656012836,21.3317331513213,73.5));
#98843=CARTESIAN_POINT('Origin',(110.,18.,73.5));
#98844=CARTESIAN_POINT('Origin',(119.934939765309,20.7548996097291,81.));
#98845=CARTESIAN_POINT('',(119.130142556433,20.9665631459995,81.));
#98846=CARTESIAN_POINT('',(119.58628655942,20.8465962131424,73.5));
#98847=CARTESIAN_POINT('Origin',(119.130142556433,20.9665631459995,81.));
#98848=CARTESIAN_POINT('Origin',(110.,18.,73.5));
#98849=CARTESIAN_POINT('',(119.833771504544,19.815747228118,73.5));
#98850=CARTESIAN_POINT('Origin',(119.481808069713,19.5017708643862,81.));
#98851=CARTESIAN_POINT('',(119.481808069713,19.5017708643862,81.));
#98852=CARTESIAN_POINT('Origin',(120.243585417398,19.1668152366466,81.));
#98853=CARTESIAN_POINT('',(119.913569220132,19.3119242804578,73.5));
#98854=CARTESIAN_POINT('Origin',(119.6,18.,81.));
#98855=CARTESIAN_POINT('',(119.6,18.,81.));
#98856=CARTESIAN_POINT('',(119.996746905394,18.2550515820388,73.5));
#98857=CARTESIAN_POINT('Origin',(120.3,17.55,81.));
#98858=CARTESIAN_POINT('Origin',(110.,18.,49.85));
#98859=CARTESIAN_POINT('',(107.49,18.,50.));
#98860=CARTESIAN_POINT('Origin',(110.,18.,50.));
#98861=CARTESIAN_POINT('',(107.19,18.,49.7));
#98862=CARTESIAN_POINT('',(107.34,18.,49.85));
#98863=CARTESIAN_POINT('Origin',(110.,18.,49.7));
#98864=CARTESIAN_POINT('Origin',(113.7,18.,49.7));
#98865=CARTESIAN_POINT('',(106.3,18.,49.7));
#98866=CARTESIAN_POINT('Origin',(110.,18.,49.7));
#98867=CARTESIAN_POINT('Origin',(110.,18.,49.85));
#98868=CARTESIAN_POINT('',(106.,18.,50.));
#98869=CARTESIAN_POINT('Origin',(110.,18.,50.));
#98870=CARTESIAN_POINT('',(106.15,18.,49.85));
#98871=CARTESIAN_POINT('Origin',(110.,18.,54.8));
#98872=CARTESIAN_POINT('',(106.,18.,59.6));
#98873=CARTESIAN_POINT('Origin',(110.,18.,59.6));
#98874=CARTESIAN_POINT('',(106.,18.,54.8));
#98875=CARTESIAN_POINT('Origin',(110.,18.,59.8));
#98876=CARTESIAN_POINT('',(105.6,18.,60.));
#98877=CARTESIAN_POINT('Origin',(110.,18.,60.));
#98878=CARTESIAN_POINT('',(105.8,18.,59.8));
#98879=CARTESIAN_POINT('Origin',(116.,18.,60.));
#98880=CARTESIAN_POINT('',(104.,18.,60.));
#98881=CARTESIAN_POINT('Origin',(110.,18.,60.));
#98882=CARTESIAN_POINT('Origin',(110.,18.,62.8));
#98883=CARTESIAN_POINT('',(104.,18.,65.6));
#98884=CARTESIAN_POINT('Origin',(110.,18.,65.6));
#98885=CARTESIAN_POINT('',(104.,18.,62.8));
#98886=CARTESIAN_POINT('Origin',(110.,18.,65.8));
#98887=CARTESIAN_POINT('',(103.6,18.,66.));
#98888=CARTESIAN_POINT('Origin',(110.,18.,66.));
#98889=CARTESIAN_POINT('',(103.8,18.,65.8));
#98890=CARTESIAN_POINT('Origin',(119.2,18.,66.));
#98891=CARTESIAN_POINT('Origin',(110.,18.,73.5));
#98892=CARTESIAN_POINT('Origin',(117.4,18.,81.));
#98893=CARTESIAN_POINT('',(102.6,18.,81.));
#98894=CARTESIAN_POINT('Origin',(110.,18.,81.));
#98895=CARTESIAN_POINT('Origin',(110.,18.,80.8));
#98896=CARTESIAN_POINT('',(103.,18.,80.6));
#98897=CARTESIAN_POINT('',(102.8,18.,80.8));
#98898=CARTESIAN_POINT('Origin',(110.,18.,80.6));
#98899=CARTESIAN_POINT('Origin',(110.,18.,80.6));
#98900=CARTESIAN_POINT('Origin',(110.,18.,78.85));
#98901=CARTESIAN_POINT('',(110.,18.,79.6));
#98902=CARTESIAN_POINT('',(107.49,18.,78.1));
#98903=CARTESIAN_POINT('',(108.745,18.,78.85));
#98904=CARTESIAN_POINT('Origin',(110.,18.,78.1));
#98905=CARTESIAN_POINT('Origin',(110.,18.,64.05));
#98906=CARTESIAN_POINT('',(107.49,18.,64.05));
#113951=UNCERTAINTY_MEASURE_WITH_UNIT(LENGTH_MEASURE(0.01),#113985,
'DISTANCE_ACCURACY_VALUE',
'Maximum model space distance between geometric entities at asserted c
onnectivities');
#113964=UNCERTAINTY_MEASURE_WITH_UNIT(LENGTH_MEASURE(0.01),#113985,
'DISTANCE_ACCURACY_VALUE',
'Maximum model space distance between geometric entities at asserted c
onnectivities');
#113971=(
GEOMETRIC_REPRESENTATION_CONTEXT(3)
GLOBAL_UNCERTAINTY_ASSIGNED_CONTEXT((#113951))
GLOBAL_UNIT_ASSIGNED_CONTEXT((#113985,#113987,#113988))
REPRESENTATION_CONTEXT('','3D')
);
#113984=(
GEOMETRIC_REPRESENTATION_CONTEXT(3)
GLOBAL_UNCERTAINTY_ASSIGNED_CONTEXT((#113964))
GLOBAL_UNIT_ASSIGNED_CONTEXT((#113985,#113987,#113988))
REPRESENTATION_CONTEXT('','3D')
);
#113985=(
LENGTH_UNIT()
NAMED_UNIT(*)
SI_UNIT(.MILLI.,.METRE.)
);
#113987=(
NAMED_UNIT(*)
PLANE_ANGLE_UNIT()
SI_UNIT($,.RADIAN.)
);
#113988=(
NAMED_UNIT(*)
SI_UNIT($,.STERADIAN.)
SOLID_ANGLE_UNIT()
);
#113995=SHAPE_DEFINITION_REPRESENTATION(#114014,#114057);
#114014=PRODUCT_DEFINITION_SHAPE('',$,#114077);
#114057=SHAPE_REPRESENTATION('',(#62138),#113971);
#114070=PRODUCT_DEFINITION_CONTEXT('part definition',#114129,'design');
#114077=PRODUCT_DEFINITION('2026-10-05-09-49-16-336',
'Knurled Adjustment Knob D20',#114096,#114070);
#114096=PRODUCT_DEFINITION_FORMATION('',$,#114137);
#114129=APPLICATION_CONTEXT(
'Core Data for Automotive Mechanical Design Process');
#114130=PRODUCT_CONTEXT('part definition',#114129,'mechanical');
#114137=PRODUCT('2026-10-05-09-49-16-336','Knurled Adjustment Knob D20',
$,(#114130));
#114318=COLOUR_RGB('Off White',0.89,0.88,0.83);
#114319=FILL_AREA_STYLE_COLOUR('',#114318);
#114320=FILL_AREA_STYLE('',(#114319));
#114321=SURFACE_STYLE_FILL_AREA(#114320);
#114322=SURFACE_SIDE_STYLE('',(#114321));
#114323=SURFACE_STYLE_USAGE(.BOTH.,#114322);
#114324=PRESENTATION_STYLE_ASSIGNMENT((#114323));
ENDSEC;
END-ISO-10303-21;
